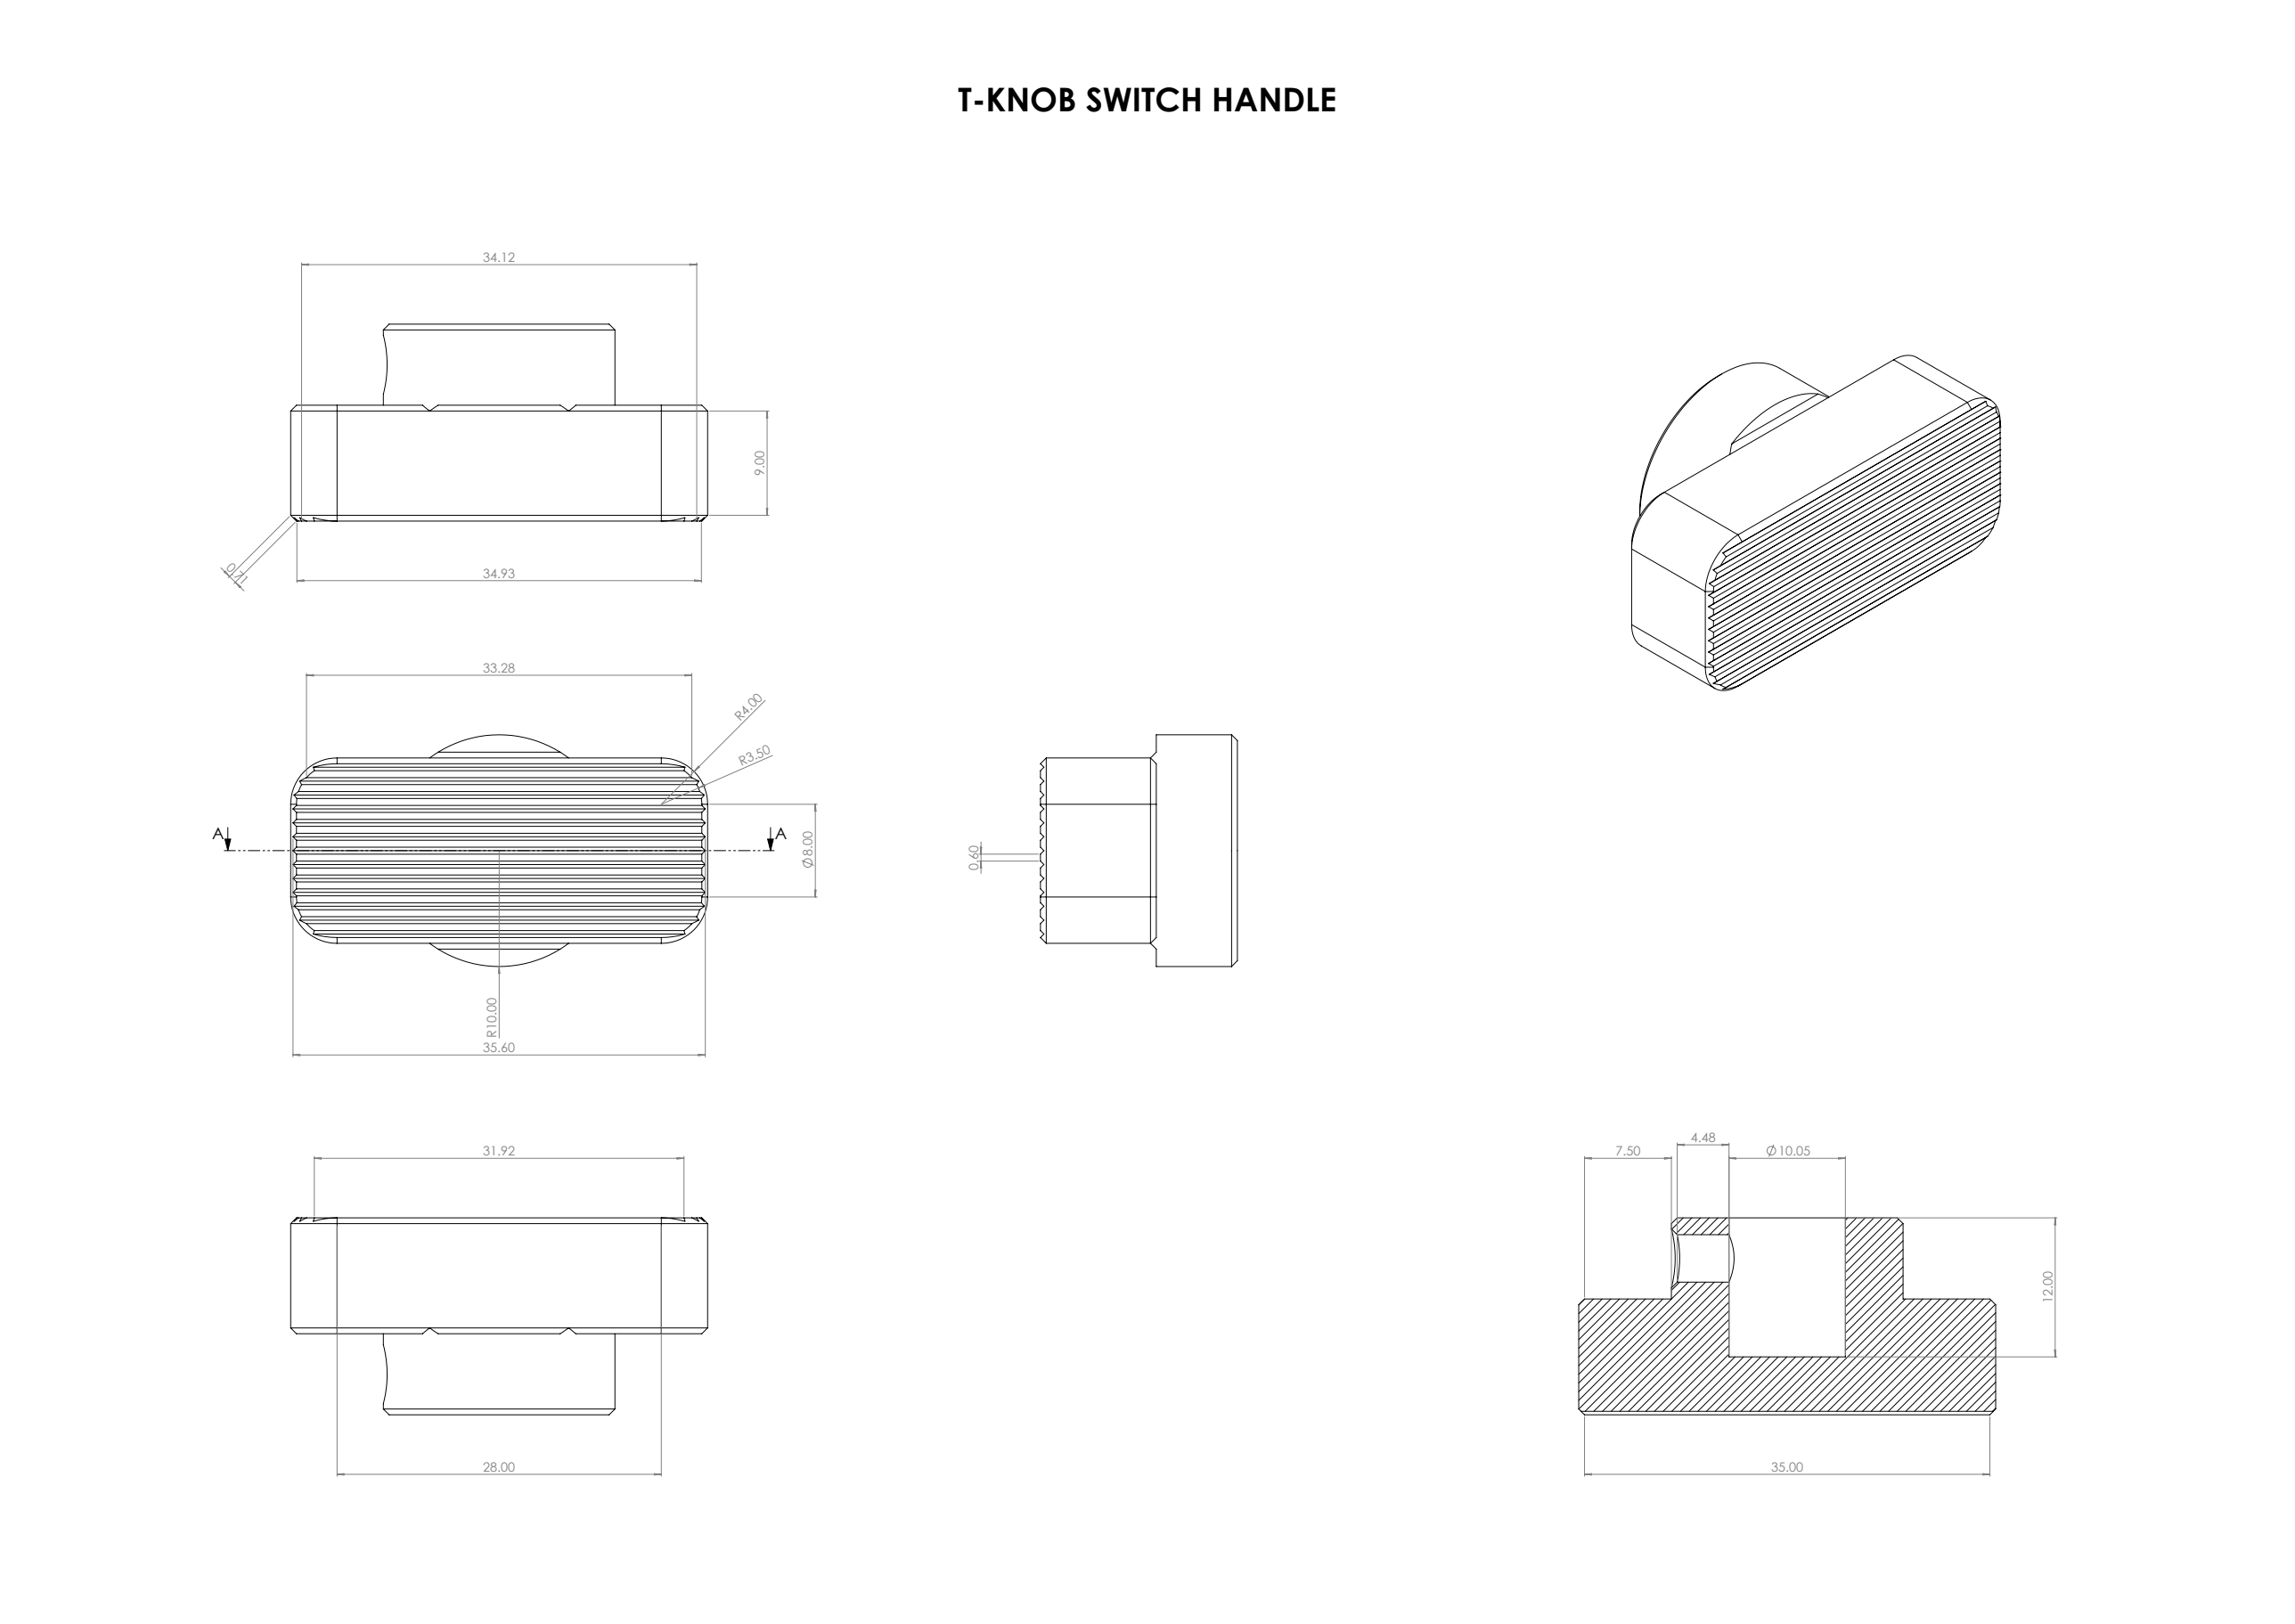
ISO-10303-21;
HEADER;
/* Generated by software containing ST-Developer
 * from STEP Tools, Inc. (www.steptools.com) 
 */

FILE_DESCRIPTION(
/* description */ (''),
/* implementation_level */ '2;1');

FILE_NAME(
/* name */ '09_T-Knob_Switch_Handle.step',
/* time_stamp */ '2026-10-21T01:59:45-07:00',
/* author */ (''),
/* organization */ (''),
/* preprocessor_version */ 'ST-DEVELOPER v20.2',
/* originating_system */ 'Autodesk Translation Framework v15.15.0.0',
/* authorisation */ '');

FILE_SCHEMA (('AUTOMOTIVE_DESIGN { 1 0 10303 214 3 1 1 }'));
ENDSEC;

DATA;
#10=MECHANICAL_DESIGN_GEOMETRIC_PRESENTATION_REPRESENTATION('',(#477),#18281);
#119=(
BOUNDED_CURVE()
B_SPLINE_CURVE(2,(#14814,#14815,#14816),.UNSPECIFIED.,.F.,.F.)
B_SPLINE_CURVE_WITH_KNOTS((3,3),(0.,0.0729284032695322),.UNSPECIFIED.)
CURVE()
GEOMETRIC_REPRESENTATION_ITEM()
RATIONAL_B_SPLINE_CURVE((1.,1.,1.))
REPRESENTATION_ITEM('')
);
#120=(
BOUNDED_CURVE()
B_SPLINE_CURVE(2,(#14820,#14821,#14822),.UNSPECIFIED.,.F.,.F.)
B_SPLINE_CURVE_WITH_KNOTS((3,3),(0.,0.072928403269532),.UNSPECIFIED.)
CURVE()
GEOMETRIC_REPRESENTATION_ITEM()
RATIONAL_B_SPLINE_CURVE((1.,1.,1.))
REPRESENTATION_ITEM('')
);
#121=(
BOUNDED_CURVE()
B_SPLINE_CURVE(2,(#14826,#14827,#14828),.UNSPECIFIED.,.F.,.F.)
B_SPLINE_CURVE_WITH_KNOTS((3,3),(0.,0.0457691166614135),.UNSPECIFIED.)
CURVE()
GEOMETRIC_REPRESENTATION_ITEM()
RATIONAL_B_SPLINE_CURVE((1.,1.,1.))
REPRESENTATION_ITEM('')
);
#122=(
BOUNDED_CURVE()
B_SPLINE_CURVE(2,(#14831,#14832,#14833),.UNSPECIFIED.,.F.,.F.)
B_SPLINE_CURVE_WITH_KNOTS((3,3),(0.,0.0457691166614134),.UNSPECIFIED.)
CURVE()
GEOMETRIC_REPRESENTATION_ITEM()
RATIONAL_B_SPLINE_CURVE((1.,1.,1.))
REPRESENTATION_ITEM('')
);
#123=(
BOUNDED_CURVE()
B_SPLINE_CURVE(2,(#14897,#14898,#14899),.UNSPECIFIED.,.F.,.F.)
B_SPLINE_CURVE_WITH_KNOTS((3,3),(0.,0.0577818255968905),.UNSPECIFIED.)
CURVE()
GEOMETRIC_REPRESENTATION_ITEM()
RATIONAL_B_SPLINE_CURVE((1.,1.,1.))
REPRESENTATION_ITEM('')
);
#124=(
BOUNDED_CURVE()
B_SPLINE_CURVE(2,(#14903,#14904,#14905),.UNSPECIFIED.,.F.,.F.)
B_SPLINE_CURVE_WITH_KNOTS((3,3),(0.,0.0577818255968905),.UNSPECIFIED.)
CURVE()
GEOMETRIC_REPRESENTATION_ITEM()
RATIONAL_B_SPLINE_CURVE((1.,1.,1.))
REPRESENTATION_ITEM('')
);
#125=(
BOUNDED_CURVE()
B_SPLINE_CURVE(2,(#14909,#14910,#14911),.UNSPECIFIED.,.F.,.F.)
B_SPLINE_CURVE_WITH_KNOTS((3,3),(0.,0.0492830096737056),.UNSPECIFIED.)
CURVE()
GEOMETRIC_REPRESENTATION_ITEM()
RATIONAL_B_SPLINE_CURVE((1.,1.,1.))
REPRESENTATION_ITEM('')
);
#126=(
BOUNDED_CURVE()
B_SPLINE_CURVE(2,(#14914,#14915,#14916),.UNSPECIFIED.,.F.,.F.)
B_SPLINE_CURVE_WITH_KNOTS((3,3),(0.,0.0492830096737056),.UNSPECIFIED.)
CURVE()
GEOMETRIC_REPRESENTATION_ITEM()
RATIONAL_B_SPLINE_CURVE((1.,1.,1.))
REPRESENTATION_ITEM('')
);
#127=(
BOUNDED_CURVE()
B_SPLINE_CURVE(2,(#14920,#14921,#14922),.UNSPECIFIED.,.F.,.F.)
B_SPLINE_CURVE_WITH_KNOTS((3,3),(0.,0.072928403269532),.UNSPECIFIED.)
CURVE()
GEOMETRIC_REPRESENTATION_ITEM()
RATIONAL_B_SPLINE_CURVE((1.,1.,1.))
REPRESENTATION_ITEM('')
);
#128=(
BOUNDED_CURVE()
B_SPLINE_CURVE(2,(#14926,#14927,#14928),.UNSPECIFIED.,.F.,.F.)
B_SPLINE_CURVE_WITH_KNOTS((3,3),(0.,0.0729284032695322),.UNSPECIFIED.)
CURVE()
GEOMETRIC_REPRESENTATION_ITEM()
RATIONAL_B_SPLINE_CURVE((1.,1.,1.))
REPRESENTATION_ITEM('')
);
#129=(
BOUNDED_CURVE()
B_SPLINE_CURVE(2,(#14932,#14933,#14934),.UNSPECIFIED.,.F.,.F.)
B_SPLINE_CURVE_WITH_KNOTS((3,3),(0.,0.0457691166614135),.UNSPECIFIED.)
CURVE()
GEOMETRIC_REPRESENTATION_ITEM()
RATIONAL_B_SPLINE_CURVE((1.,1.,1.))
REPRESENTATION_ITEM('')
);
#130=(
BOUNDED_CURVE()
B_SPLINE_CURVE(2,(#14937,#14938,#14939),.UNSPECIFIED.,.F.,.F.)
B_SPLINE_CURVE_WITH_KNOTS((3,3),(0.,0.0457691166614134),.UNSPECIFIED.)
CURVE()
GEOMETRIC_REPRESENTATION_ITEM()
RATIONAL_B_SPLINE_CURVE((1.,1.,1.))
REPRESENTATION_ITEM('')
);
#131=(
BOUNDED_CURVE()
B_SPLINE_CURVE(2,(#14973,#14974,#14975),.UNSPECIFIED.,.F.,.F.)
B_SPLINE_CURVE_WITH_KNOTS((3,3),(0.,0.210313307559557),.UNSPECIFIED.)
CURVE()
GEOMETRIC_REPRESENTATION_ITEM()
RATIONAL_B_SPLINE_CURVE((1.,1.,1.))
REPRESENTATION_ITEM('')
);
#132=(
BOUNDED_CURVE()
B_SPLINE_CURVE(2,(#14979,#14980,#14981),.UNSPECIFIED.,.F.,.F.)
B_SPLINE_CURVE_WITH_KNOTS((3,3),(0.210313307559557,0.420626615119114),
 .UNSPECIFIED.)
CURVE()
GEOMETRIC_REPRESENTATION_ITEM()
RATIONAL_B_SPLINE_CURVE((1.,1.,1.))
REPRESENTATION_ITEM('')
);
#133=(
BOUNDED_CURVE()
B_SPLINE_CURVE(2,(#14985,#14986,#14987),.UNSPECIFIED.,.F.,.F.)
B_SPLINE_CURVE_WITH_KNOTS((3,3),(0.,0.0433664286594662),.UNSPECIFIED.)
CURVE()
GEOMETRIC_REPRESENTATION_ITEM()
RATIONAL_B_SPLINE_CURVE((1.,1.,1.))
REPRESENTATION_ITEM('')
);
#134=(
BOUNDED_CURVE()
B_SPLINE_CURVE(2,(#14990,#14991,#14992),.UNSPECIFIED.,.F.,.F.)
B_SPLINE_CURVE_WITH_KNOTS((3,3),(0.,0.0433664286594663),.UNSPECIFIED.)
CURVE()
GEOMETRIC_REPRESENTATION_ITEM()
RATIONAL_B_SPLINE_CURVE((1.,1.,1.))
REPRESENTATION_ITEM('')
);
#135=(
BOUNDED_CURVE()
B_SPLINE_CURVE(2,(#15011,#15012,#15013),.UNSPECIFIED.,.F.,.F.)
B_SPLINE_CURVE_WITH_KNOTS((3,3),(0.,0.0577818255968905),.UNSPECIFIED.)
CURVE()
GEOMETRIC_REPRESENTATION_ITEM()
RATIONAL_B_SPLINE_CURVE((1.,1.,1.))
REPRESENTATION_ITEM('')
);
#136=(
BOUNDED_CURVE()
B_SPLINE_CURVE(2,(#15017,#15018,#15019),.UNSPECIFIED.,.F.,.F.)
B_SPLINE_CURVE_WITH_KNOTS((3,3),(0.,0.0577818255968905),.UNSPECIFIED.)
CURVE()
GEOMETRIC_REPRESENTATION_ITEM()
RATIONAL_B_SPLINE_CURVE((1.,1.,1.))
REPRESENTATION_ITEM('')
);
#137=(
BOUNDED_CURVE()
B_SPLINE_CURVE(2,(#15023,#15024,#15025),.UNSPECIFIED.,.F.,.F.)
B_SPLINE_CURVE_WITH_KNOTS((3,3),(0.,0.0492830096737056),.UNSPECIFIED.)
CURVE()
GEOMETRIC_REPRESENTATION_ITEM()
RATIONAL_B_SPLINE_CURVE((1.,1.,1.))
REPRESENTATION_ITEM('')
);
#138=(
BOUNDED_CURVE()
B_SPLINE_CURVE(2,(#15028,#15029,#15030),.UNSPECIFIED.,.F.,.F.)
B_SPLINE_CURVE_WITH_KNOTS((3,3),(0.,0.0492830096737056),.UNSPECIFIED.)
CURVE()
GEOMETRIC_REPRESENTATION_ITEM()
RATIONAL_B_SPLINE_CURVE((1.,1.,1.))
REPRESENTATION_ITEM('')
);
#139=(
BOUNDED_CURVE()
B_SPLINE_CURVE(2,(#15034,#15035,#15036),.UNSPECIFIED.,.F.,.F.)
B_SPLINE_CURVE_WITH_KNOTS((3,3),(0.,0.0433664286594662),.UNSPECIFIED.)
CURVE()
GEOMETRIC_REPRESENTATION_ITEM()
RATIONAL_B_SPLINE_CURVE((1.,1.,1.))
REPRESENTATION_ITEM('')
);
#140=(
BOUNDED_CURVE()
B_SPLINE_CURVE(2,(#15040,#15041,#15042),.UNSPECIFIED.,.F.,.F.)
B_SPLINE_CURVE_WITH_KNOTS((3,3),(0.,0.0433664286594662),.UNSPECIFIED.)
CURVE()
GEOMETRIC_REPRESENTATION_ITEM()
RATIONAL_B_SPLINE_CURVE((1.,1.,1.))
REPRESENTATION_ITEM('')
);
#141=(
BOUNDED_CURVE()
B_SPLINE_CURVE(2,(#15046,#15047,#15048),.UNSPECIFIED.,.F.,.F.)
B_SPLINE_CURVE_WITH_KNOTS((3,3),(0.210313307559558,0.420626615119116),
 .UNSPECIFIED.)
CURVE()
GEOMETRIC_REPRESENTATION_ITEM()
RATIONAL_B_SPLINE_CURVE((1.,1.,1.))
REPRESENTATION_ITEM('')
);
#142=(
BOUNDED_CURVE()
B_SPLINE_CURVE(2,(#15051,#15052,#15053),.UNSPECIFIED.,.F.,.F.)
B_SPLINE_CURVE_WITH_KNOTS((3,3),(0.,0.210313307559558),.UNSPECIFIED.)
CURVE()
GEOMETRIC_REPRESENTATION_ITEM()
RATIONAL_B_SPLINE_CURVE((1.,1.,1.))
REPRESENTATION_ITEM('')
);
#183=B_SPLINE_SURFACE_WITH_KNOTS('',3,3,((#14625,#14626,#14627,#14628,#14629,
#14630,#14631,#14632,#14633,#14634,#14635,#14636,#14637,#14638,#14639,#14640,
#14641,#14642,#14643,#14644),(#14645,#14646,#14647,#14648,#14649,#14650,
#14651,#14652,#14653,#14654,#14655,#14656,#14657,#14658,#14659,#14660,#14661,
#14662,#14663,#14664),(#14665,#14666,#14667,#14668,#14669,#14670,#14671,
#14672,#14673,#14674,#14675,#14676,#14677,#14678,#14679,#14680,#14681,#14682,
#14683,#14684),(#14685,#14686,#14687,#14688,#14689,#14690,#14691,#14692,
#14693,#14694,#14695,#14696,#14697,#14698,#14699,#14700,#14701,#14702,#14703,
#14704)),.UNSPECIFIED.,.F.,.T.,.F.,(4,4),(4,1,1,1,1,1,1,1,1,1,1,1,1,1,1,
1,1,4),(0.,1.),(0.929489890414013,1.01801273712011,1.06227416047316,1.10653558382621,
1.1950584305323,1.2835812772384,1.3721041239445,1.41636554729754,1.46062697065059,
1.54914981735669,1.63767266406279,1.68193408741583,1.72619551076888,1.81471835747498,
1.90324120418107,1.99176405088717,2.08028689759327,2.16880974429936),
 .UNSPECIFIED.);
#281=B_SPLINE_CURVE_WITH_KNOTS('',3,(#14708,#14709,#14710,#14711,#14712,
#14713,#14714,#14715,#14716,#14717,#14718,#14719,#14720,#14721,#14722,#14723,
#14724,#14725,#14726,#14727),.UNSPECIFIED.,.T.,.F.,(4,1,1,1,1,1,1,1,1,1,
1,1,1,1,1,1,1,4),(0.929489890414013,1.01801273712011,1.06227416047316,1.10653558382621,
1.1950584305323,1.2835812772384,1.3721041239445,1.41636554729754,1.46062697065059,
1.54914981735669,1.63767266406279,1.68193408741583,1.72619551076888,1.81471835747498,
1.90324120418107,1.99176405088717,2.08028689759327,2.16880974429936),
 .UNSPECIFIED.);
#282=B_SPLINE_CURVE_WITH_KNOTS('',3,(#14728,#14729,#14730,#14731,#14732,
#14733,#14734,#14735,#14736,#14737,#14738,#14739,#14740,#14741,#14742,#14743,
#14744,#14745,#14746,#14747),.UNSPECIFIED.,.T.,.F.,(4,1,1,1,1,1,1,1,1,1,
1,1,1,1,1,1,1,4),(-2.16880974429936,-2.08028689759327,-1.99176405088717,
-1.90324120418107,-1.81471835747498,-1.72619551076888,-1.68193408741583,
-1.63767266406279,-1.54914981735669,-1.46062697065059,-1.41636554729754,
-1.3721041239445,-1.2835812772384,-1.1950584305323,-1.10653558382621,-1.06227416047316,
-1.01801273712011,-0.929489890414013),.UNSPECIFIED.);
#283=B_SPLINE_CURVE_WITH_KNOTS('',3,(#14752,#14753,#14754,#14755,#14756,
#14757,#14758,#14759,#14760,#14761),.UNSPECIFIED.,.F.,.F.,(4,2,2,2,4),(0.,
0.0782650235733475,0.156530047146695,0.234708817404274,0.312887587661852),
 .UNSPECIFIED.);
#284=B_SPLINE_CURVE_WITH_KNOTS('',3,(#14762,#14763,#14764,#14765,#14766,
#14767,#14768,#14769,#14770,#14771,#14772,#14773,#14774,#14775,#14776,#14777,
#14778,#14779,#14780,#14781,#14782,#14783,#14784,#14785,#14786,#14787),
 .UNSPECIFIED.,.F.,.F.,(4,2,2,2,2,2,2,2,2,2,2,2,4),(0.312887587661852,0.391066357919431,
0.469245128177009,0.547510151750357,0.625775175323705,0.704040198897052,
0.782305222470399,0.860483992727978,0.938662762985557,1.01684153324314,
1.09502030350071,1.17328532707406,1.25155035064741),.UNSPECIFIED.);
#421=CONICAL_SURFACE('',#9730,3.75,0.785398163397447);
#422=CONICAL_SURFACE('',#9738,3.75,0.785398163397447);
#423=CONICAL_SURFACE('',#9741,3.75,0.785398163397447);
#424=CONICAL_SURFACE('',#9748,3.75,0.785398163397447);
#425=CONICAL_SURFACE('',#9792,3.75,0.785398163397448);
#426=CONICAL_SURFACE('',#9816,3.75,0.785398163397447);
#427=CONICAL_SURFACE('',#9831,3.75,0.785398163397447);
#428=CONICAL_SURFACE('',#9834,3.75,0.785398163397448);
#429=CONICAL_SURFACE('',#9846,9.75,0.785398163397449);
#446=SHAPE_REPRESENTATION_RELATIONSHIP('SRR','None',#18348,#459);
#459=ADVANCED_BREP_SHAPE_REPRESENTATION('',(#490),#18277);
#477=STYLED_ITEM('',(#18488),#490);
#490=MANIFOLD_SOLID_BREP('Body1',#9094);
#533=CYLINDRICAL_SURFACE('',#9752,2.05);
#534=CYLINDRICAL_SURFACE('',#9753,10.);
#535=CYLINDRICAL_SURFACE('',#9823,4.);
#536=CYLINDRICAL_SURFACE('',#9825,4.);
#537=CYLINDRICAL_SURFACE('',#9828,4.);
#538=CYLINDRICAL_SURFACE('',#9838,4.);
#539=CYLINDRICAL_SURFACE('',#9842,5.025);
#623=FACE_BOUND('',#1792,.T.);
#624=FACE_BOUND('',#1855,.T.);
#625=FACE_BOUND('',#1857,.T.);
#763=CIRCLE('',#9731,4.);
#764=CIRCLE('',#9732,3.5);
#765=CIRCLE('',#9736,3.5);
#766=CIRCLE('',#9737,10.);
#767=CIRCLE('',#9739,4.);
#768=CIRCLE('',#9742,4.);
#769=CIRCLE('',#9743,3.5);
#770=CIRCLE('',#9746,10.);
#771=CIRCLE('',#9747,3.5);
#772=CIRCLE('',#9749,4.);
#773=CIRCLE('',#9757,10.);
#774=CIRCLE('',#9758,10.);
#775=CIRCLE('',#9759,10.);
#776=CIRCLE('',#9763,10.);
#777=CIRCLE('',#9765,5.025);
#778=CIRCLE('',#9793,3.5);
#779=CIRCLE('',#9794,4.);
#780=CIRCLE('',#9795,3.5);
#781=CIRCLE('',#9796,3.5);
#782=CIRCLE('',#9799,3.5);
#783=CIRCLE('',#9800,3.5);
#784=CIRCLE('',#9802,3.5);
#785=CIRCLE('',#9803,3.5);
#786=CIRCLE('',#9807,3.5);
#787=CIRCLE('',#9809,3.5);
#788=CIRCLE('',#9811,3.5);
#789=CIRCLE('',#9817,4.);
#790=CIRCLE('',#9818,3.5);
#791=CIRCLE('',#9826,4.);
#792=CIRCLE('',#9829,4.);
#793=CIRCLE('',#9835,3.5);
#794=CIRCLE('',#9843,5.025);
#795=CIRCLE('',#9845,9.5);
#834=ELLIPSE('',#9734,14.142135623731,10.);
#835=ELLIPSE('',#9751,14.142135623731,10.);
#836=ELLIPSE('',#9754,14.142135623731,10.);
#837=ELLIPSE('',#9755,14.142135623731,10.);
#838=ELLIPSE('',#9756,14.142135623731,10.);
#839=ELLIPSE('',#9760,14.142135623731,10.);
#840=ELLIPSE('',#9761,14.142135623731,10.);
#841=ELLIPSE('',#9762,14.142135623731,10.);
#1213=FACE_OUTER_BOUND('',#1779,.T.);
#1214=FACE_OUTER_BOUND('',#1780,.T.);
#1215=FACE_OUTER_BOUND('',#1781,.T.);
#1216=FACE_OUTER_BOUND('',#1782,.T.);
#1217=FACE_OUTER_BOUND('',#1783,.T.);
#1218=FACE_OUTER_BOUND('',#1784,.T.);
#1219=FACE_OUTER_BOUND('',#1785,.T.);
#1220=FACE_OUTER_BOUND('',#1786,.T.);
#1221=FACE_OUTER_BOUND('',#1787,.T.);
#1222=FACE_OUTER_BOUND('',#1788,.T.);
#1223=FACE_OUTER_BOUND('',#1789,.T.);
#1224=FACE_OUTER_BOUND('',#1790,.T.);
#1225=FACE_OUTER_BOUND('',#1791,.T.);
#1226=FACE_OUTER_BOUND('',#1793,.T.);
#1227=FACE_OUTER_BOUND('',#1794,.T.);
#1228=FACE_OUTER_BOUND('',#1795,.T.);
#1229=FACE_OUTER_BOUND('',#1796,.T.);
#1230=FACE_OUTER_BOUND('',#1797,.T.);
#1231=FACE_OUTER_BOUND('',#1798,.T.);
#1232=FACE_OUTER_BOUND('',#1799,.T.);
#1233=FACE_OUTER_BOUND('',#1800,.T.);
#1234=FACE_OUTER_BOUND('',#1801,.T.);
#1235=FACE_OUTER_BOUND('',#1802,.T.);
#1236=FACE_OUTER_BOUND('',#1803,.T.);
#1237=FACE_OUTER_BOUND('',#1804,.T.);
#1238=FACE_OUTER_BOUND('',#1805,.T.);
#1239=FACE_OUTER_BOUND('',#1806,.T.);
#1240=FACE_OUTER_BOUND('',#1807,.T.);
#1241=FACE_OUTER_BOUND('',#1808,.T.);
#1242=FACE_OUTER_BOUND('',#1809,.T.);
#1243=FACE_OUTER_BOUND('',#1810,.T.);
#1244=FACE_OUTER_BOUND('',#1811,.T.);
#1245=FACE_OUTER_BOUND('',#1812,.T.);
#1246=FACE_OUTER_BOUND('',#1813,.T.);
#1247=FACE_OUTER_BOUND('',#1814,.T.);
#1248=FACE_OUTER_BOUND('',#1815,.T.);
#1249=FACE_OUTER_BOUND('',#1816,.T.);
#1250=FACE_OUTER_BOUND('',#1817,.T.);
#1251=FACE_OUTER_BOUND('',#1818,.T.);
#1252=FACE_OUTER_BOUND('',#1819,.T.);
#1253=FACE_OUTER_BOUND('',#1820,.T.);
#1254=FACE_OUTER_BOUND('',#1821,.T.);
#1255=FACE_OUTER_BOUND('',#1822,.T.);
#1256=FACE_OUTER_BOUND('',#1823,.T.);
#1257=FACE_OUTER_BOUND('',#1824,.T.);
#1258=FACE_OUTER_BOUND('',#1825,.T.);
#1259=FACE_OUTER_BOUND('',#1826,.T.);
#1260=FACE_OUTER_BOUND('',#1827,.T.);
#1261=FACE_OUTER_BOUND('',#1828,.T.);
#1262=FACE_OUTER_BOUND('',#1829,.T.);
#1263=FACE_OUTER_BOUND('',#1830,.T.);
#1264=FACE_OUTER_BOUND('',#1831,.T.);
#1265=FACE_OUTER_BOUND('',#1832,.T.);
#1266=FACE_OUTER_BOUND('',#1833,.T.);
#1267=FACE_OUTER_BOUND('',#1834,.T.);
#1268=FACE_OUTER_BOUND('',#1835,.T.);
#1269=FACE_OUTER_BOUND('',#1836,.T.);
#1270=FACE_OUTER_BOUND('',#1837,.T.);
#1271=FACE_OUTER_BOUND('',#1838,.T.);
#1272=FACE_OUTER_BOUND('',#1839,.T.);
#1273=FACE_OUTER_BOUND('',#1840,.T.);
#1274=FACE_OUTER_BOUND('',#1841,.T.);
#1275=FACE_OUTER_BOUND('',#1842,.T.);
#1276=FACE_OUTER_BOUND('',#1843,.T.);
#1277=FACE_OUTER_BOUND('',#1844,.T.);
#1278=FACE_OUTER_BOUND('',#1845,.T.);
#1279=FACE_OUTER_BOUND('',#1846,.T.);
#1280=FACE_OUTER_BOUND('',#1847,.T.);
#1281=FACE_OUTER_BOUND('',#1848,.T.);
#1282=FACE_OUTER_BOUND('',#1849,.T.);
#1283=FACE_OUTER_BOUND('',#1850,.T.);
#1284=FACE_OUTER_BOUND('',#1851,.T.);
#1285=FACE_OUTER_BOUND('',#1852,.T.);
#1286=FACE_OUTER_BOUND('',#1853,.T.);
#1287=FACE_OUTER_BOUND('',#1854,.T.);
#1288=FACE_OUTER_BOUND('',#1856,.T.);
#1289=FACE_OUTER_BOUND('',#1858,.T.);
#1779=EDGE_LOOP('',(#7464,#7465,#7466,#7467));
#1780=EDGE_LOOP('',(#7468,#7469,#7470,#7471));
#1781=EDGE_LOOP('',(#7472,#7473,#7474,#7475,#7476,#7477));
#1782=EDGE_LOOP('',(#7478,#7479,#7480,#7481));
#1783=EDGE_LOOP('',(#7482,#7483,#7484,#7485));
#1784=EDGE_LOOP('',(#7486,#7487,#7488,#7489));
#1785=EDGE_LOOP('',(#7490,#7491,#7492,#7493));
#1786=EDGE_LOOP('',(#7494,#7495,#7496,#7497,#7498,#7499));
#1787=EDGE_LOOP('',(#7500,#7501,#7502,#7503));
#1788=EDGE_LOOP('',(#7504,#7505,#7506,#7507));
#1789=EDGE_LOOP('',(#7508,#7509,#7510,#7511));
#1790=EDGE_LOOP('',(#7512,#7513,#7514,#7515,#7516));
#1791=EDGE_LOOP('',(#7517,#7518,#7519,#7520,#7521,#7522,#7523,#7524,#7525,
#7526,#7527,#7528,#7529,#7530,#7531,#7532));
#1792=EDGE_LOOP('',(#7533));
#1793=EDGE_LOOP('',(#7534));
#1794=EDGE_LOOP('',(#7535,#7536,#7537,#7538));
#1795=EDGE_LOOP('',(#7539,#7540,#7541,#7542));
#1796=EDGE_LOOP('',(#7543,#7544,#7545,#7546));
#1797=EDGE_LOOP('',(#7547,#7548,#7549,#7550));
#1798=EDGE_LOOP('',(#7551,#7552,#7553,#7554));
#1799=EDGE_LOOP('',(#7555,#7556,#7557,#7558));
#1800=EDGE_LOOP('',(#7559,#7560,#7561,#7562));
#1801=EDGE_LOOP('',(#7563,#7564,#7565,#7566));
#1802=EDGE_LOOP('',(#7567,#7568,#7569,#7570));
#1803=EDGE_LOOP('',(#7571,#7572,#7573,#7574));
#1804=EDGE_LOOP('',(#7575,#7576,#7577,#7578));
#1805=EDGE_LOOP('',(#7579,#7580,#7581,#7582));
#1806=EDGE_LOOP('',(#7583,#7584,#7585,#7586));
#1807=EDGE_LOOP('',(#7587,#7588,#7589,#7590));
#1808=EDGE_LOOP('',(#7591,#7592,#7593,#7594));
#1809=EDGE_LOOP('',(#7595,#7596,#7597,#7598));
#1810=EDGE_LOOP('',(#7599,#7600,#7601,#7602));
#1811=EDGE_LOOP('',(#7603,#7604,#7605,#7606));
#1812=EDGE_LOOP('',(#7607,#7608,#7609,#7610));
#1813=EDGE_LOOP('',(#7611,#7612,#7613,#7614));
#1814=EDGE_LOOP('',(#7615,#7616,#7617,#7618));
#1815=EDGE_LOOP('',(#7619,#7620,#7621,#7622));
#1816=EDGE_LOOP('',(#7623,#7624,#7625,#7626));
#1817=EDGE_LOOP('',(#7627,#7628,#7629,#7630));
#1818=EDGE_LOOP('',(#7631,#7632,#7633,#7634));
#1819=EDGE_LOOP('',(#7635,#7636,#7637,#7638));
#1820=EDGE_LOOP('',(#7639,#7640,#7641,#7642,#7643,#7644,#7645,#7646,#7647,
#7648,#7649,#7650));
#1821=EDGE_LOOP('',(#7651,#7652,#7653,#7654,#7655,#7656,#7657,#7658,#7659,
#7660,#7661,#7662,#7663,#7664,#7665,#7666,#7667,#7668,#7669,#7670,#7671,
#7672,#7673,#7674,#7675));
#1822=EDGE_LOOP('',(#7676,#7677,#7678,#7679));
#1823=EDGE_LOOP('',(#7680,#7681,#7682,#7683,#7684,#7685));
#1824=EDGE_LOOP('',(#7686,#7687,#7688,#7689));
#1825=EDGE_LOOP('',(#7690,#7691,#7692,#7693));
#1826=EDGE_LOOP('',(#7694,#7695,#7696,#7697));
#1827=EDGE_LOOP('',(#7698,#7699,#7700,#7701));
#1828=EDGE_LOOP('',(#7702,#7703,#7704,#7705,#7706,#7707));
#1829=EDGE_LOOP('',(#7708,#7709,#7710,#7711));
#1830=EDGE_LOOP('',(#7712,#7713,#7714,#7715));
#1831=EDGE_LOOP('',(#7716,#7717,#7718,#7719));
#1832=EDGE_LOOP('',(#7720,#7721,#7722,#7723));
#1833=EDGE_LOOP('',(#7724,#7725,#7726,#7727,#7728,#7729,#7730,#7731,#7732,
#7733,#7734,#7735));
#1834=EDGE_LOOP('',(#7736,#7737,#7738,#7739));
#1835=EDGE_LOOP('',(#7740,#7741,#7742,#7743,#7744,#7745));
#1836=EDGE_LOOP('',(#7746,#7747,#7748,#7749));
#1837=EDGE_LOOP('',(#7750,#7751,#7752,#7753,#7754,#7755));
#1838=EDGE_LOOP('',(#7756,#7757,#7758,#7759));
#1839=EDGE_LOOP('',(#7760,#7761,#7762,#7763));
#1840=EDGE_LOOP('',(#7764,#7765,#7766,#7767));
#1841=EDGE_LOOP('',(#7768,#7769,#7770,#7771));
#1842=EDGE_LOOP('',(#7772,#7773,#7774,#7775));
#1843=EDGE_LOOP('',(#7776,#7777,#7778,#7779));
#1844=EDGE_LOOP('',(#7780,#7781,#7782,#7783,#7784,#7785,#7786,#7787,#7788,
#7789,#7790,#7791));
#1845=EDGE_LOOP('',(#7792,#7793,#7794,#7795));
#1846=EDGE_LOOP('',(#7796,#7797,#7798,#7799));
#1847=EDGE_LOOP('',(#7800,#7801,#7802,#7803,#7804,#7805,#7806,#7807,#7808,
#7809,#7810,#7811));
#1848=EDGE_LOOP('',(#7812,#7813,#7814,#7815,#7816,#7817,#7818,#7819,#7820,
#7821,#7822,#7823,#7824,#7825,#7826,#7827,#7828,#7829,#7830,#7831,#7832,
#7833,#7834,#7835,#7836));
#1849=EDGE_LOOP('',(#7837,#7838,#7839,#7840));
#1850=EDGE_LOOP('',(#7841,#7842,#7843,#7844));
#1851=EDGE_LOOP('',(#7845,#7846,#7847,#7848));
#1852=EDGE_LOOP('',(#7849,#7850,#7851));
#1853=EDGE_LOOP('',(#7852,#7853));
#1854=EDGE_LOOP('',(#7854,#7855,#7856,#7857));
#1855=EDGE_LOOP('',(#7858,#7859));
#1856=EDGE_LOOP('',(#7860));
#1857=EDGE_LOOP('',(#7861));
#1858=EDGE_LOOP('',(#7862,#7863,#7864,#7865));
#2571=LINE('',#14566,#3416);
#2572=LINE('',#14570,#3417);
#2573=LINE('',#14574,#3418);
#2574=LINE('',#14577,#3419);
#2575=LINE('',#14580,#3420);
#2576=LINE('',#14584,#3421);
#2577=LINE('',#14588,#3422);
#2578=LINE('',#14591,#3423);
#2579=LINE('',#14593,#3424);
#2580=LINE('',#14597,#3425);
#2581=LINE('',#14601,#3426);
#2582=LINE('',#14605,#3427);
#2583=LINE('',#14607,#3428);
#2584=LINE('',#14608,#3429);
#2585=LINE('',#14611,#3430);
#2586=LINE('',#14615,#3431);
#2587=LINE('',#14619,#3432);
#2588=LINE('',#14624,#3433);
#2589=LINE('',#14707,#3434);
#2590=LINE('',#14750,#3435);
#2591=LINE('',#14798,#3436);
#2592=LINE('',#14818,#3437);
#2593=LINE('',#14823,#3438);
#2594=LINE('',#14830,#3439);
#2595=LINE('',#14837,#3440);
#2596=LINE('',#14839,#3441);
#2597=LINE('',#14841,#3442);
#2598=LINE('',#14842,#3443);
#2599=LINE('',#14845,#3444);
#2600=LINE('',#14847,#3445);
#2601=LINE('',#14848,#3446);
#2602=LINE('',#14852,#3447);
#2603=LINE('',#14854,#3448);
#2604=LINE('',#14856,#3449);
#2605=LINE('',#14857,#3450);
#2606=LINE('',#14860,#3451);
#2607=LINE('',#14862,#3452);
#2608=LINE('',#14863,#3453);
#2609=LINE('',#14867,#3454);
#2610=LINE('',#14869,#3455);
#2611=LINE('',#14871,#3456);
#2612=LINE('',#14872,#3457);
#2613=LINE('',#14875,#3458);
#2614=LINE('',#14877,#3459);
#2615=LINE('',#14878,#3460);
#2616=LINE('',#14882,#3461);
#2617=LINE('',#14884,#3462);
#2618=LINE('',#14886,#3463);
#2619=LINE('',#14887,#3464);
#2620=LINE('',#14890,#3465);
#2621=LINE('',#14892,#3466);
#2622=LINE('',#14893,#3467);
#2623=LINE('',#14901,#3468);
#2624=LINE('',#14906,#3469);
#2625=LINE('',#14913,#3470);
#2626=LINE('',#14924,#3471);
#2627=LINE('',#14929,#3472);
#2628=LINE('',#14936,#3473);
#2629=LINE('',#14943,#3474);
#2630=LINE('',#14945,#3475);
#2631=LINE('',#14947,#3476);
#2632=LINE('',#14948,#3477);
#2633=LINE('',#14951,#3478);
#2634=LINE('',#14953,#3479);
#2635=LINE('',#14954,#3480);
#2636=LINE('',#14958,#3481);
#2637=LINE('',#14960,#3482);
#2638=LINE('',#14962,#3483);
#2639=LINE('',#14963,#3484);
#2640=LINE('',#14966,#3485);
#2641=LINE('',#14968,#3486);
#2642=LINE('',#14969,#3487);
#2643=LINE('',#14977,#3488);
#2644=LINE('',#14982,#3489);
#2645=LINE('',#14989,#3490);
#2646=LINE('',#14996,#3491);
#2647=LINE('',#14998,#3492);
#2648=LINE('',#15000,#3493);
#2649=LINE('',#15001,#3494);
#2650=LINE('',#15004,#3495);
#2651=LINE('',#15006,#3496);
#2652=LINE('',#15007,#3497);
#2653=LINE('',#15015,#3498);
#2654=LINE('',#15020,#3499);
#2655=LINE('',#15027,#3500);
#2656=LINE('',#15038,#3501);
#2657=LINE('',#15043,#3502);
#2658=LINE('',#15050,#3503);
#2659=LINE('',#15058,#3504);
#2660=LINE('',#15061,#3505);
#2661=LINE('',#15066,#3506);
#2662=LINE('',#15068,#3507);
#2663=LINE('',#15069,#3508);
#2664=LINE('',#15070,#3509);
#2665=LINE('',#15071,#3510);
#2666=LINE('',#15072,#3511);
#2667=LINE('',#15073,#3512);
#2668=LINE('',#15074,#3513);
#2669=LINE('',#15075,#3514);
#2670=LINE('',#15076,#3515);
#2671=LINE('',#15082,#3516);
#2672=LINE('',#15086,#3517);
#2673=LINE('',#15088,#3518);
#2674=LINE('',#15096,#3519);
#2675=LINE('',#15098,#3520);
#2676=LINE('',#15100,#3521);
#2677=LINE('',#15102,#3522);
#2678=LINE('',#15104,#3523);
#2679=LINE('',#15107,#3524);
#2680=LINE('',#15111,#3525);
#2681=LINE('',#15112,#3526);
#2682=LINE('',#15114,#3527);
#2683=LINE('',#15116,#3528);
#2684=LINE('',#15117,#3529);
#2685=LINE('',#15118,#3530);
#2686=LINE('',#15120,#3531);
#2687=LINE('',#15121,#3532);
#2688=LINE('',#15123,#3533);
#2689=LINE('',#15124,#3534);
#2690=LINE('',#15126,#3535);
#2691=LINE('',#15127,#3536);
#2692=LINE('',#15129,#3537);
#2693=LINE('',#15133,#3538);
#2694=LINE('',#15139,#3539);
#2695=LINE('',#15141,#3540);
#2696=LINE('',#15143,#3541);
#2697=LINE('',#15144,#3542);
#2698=LINE('',#15147,#3543);
#2699=LINE('',#15150,#3544);
#2700=LINE('',#15154,#3545);
#2701=LINE('',#15160,#3546);
#2702=LINE('',#15166,#3547);
#3416=VECTOR('',#11583,10.);
#3417=VECTOR('',#11586,10.);
#3418=VECTOR('',#11591,10.);
#3419=VECTOR('',#11594,10.);
#3420=VECTOR('',#11597,10.);
#3421=VECTOR('',#11600,10.);
#3422=VECTOR('',#11605,10.);
#3423=VECTOR('',#11608,10.);
#3424=VECTOR('',#11611,10.);
#3425=VECTOR('',#11614,10.);
#3426=VECTOR('',#11617,10.);
#3427=VECTOR('',#11622,10.);
#3428=VECTOR('',#11623,10.);
#3429=VECTOR('',#11624,10.);
#3430=VECTOR('',#11627,10.);
#3431=VECTOR('',#11630,10.);
#3432=VECTOR('',#11635,10.);
#3433=VECTOR('',#11642,10.);
#3434=VECTOR('',#11643,10.);
#3435=VECTOR('',#11646,2.05);
#3436=VECTOR('',#11657,10.);
#3437=VECTOR('',#11676,10.);
#3438=VECTOR('',#11677,10.);
#3439=VECTOR('',#11680,10.);
#3440=VECTOR('',#11683,10.);
#3441=VECTOR('',#11684,10.);
#3442=VECTOR('',#11685,10.);
#3443=VECTOR('',#11686,10.);
#3444=VECTOR('',#11689,10.);
#3445=VECTOR('',#11690,10.);
#3446=VECTOR('',#11691,10.);
#3447=VECTOR('',#11694,10.);
#3448=VECTOR('',#11695,10.);
#3449=VECTOR('',#11696,10.);
#3450=VECTOR('',#11697,10.);
#3451=VECTOR('',#11700,10.);
#3452=VECTOR('',#11701,10.);
#3453=VECTOR('',#11702,10.);
#3454=VECTOR('',#11705,10.);
#3455=VECTOR('',#11706,10.);
#3456=VECTOR('',#11707,10.);
#3457=VECTOR('',#11708,10.);
#3458=VECTOR('',#11711,10.);
#3459=VECTOR('',#11712,10.);
#3460=VECTOR('',#11713,10.);
#3461=VECTOR('',#11716,10.);
#3462=VECTOR('',#11717,10.);
#3463=VECTOR('',#11718,10.);
#3464=VECTOR('',#11719,10.);
#3465=VECTOR('',#11722,10.);
#3466=VECTOR('',#11723,10.);
#3467=VECTOR('',#11724,10.);
#3468=VECTOR('',#11727,10.);
#3469=VECTOR('',#11728,10.);
#3470=VECTOR('',#11731,10.);
#3471=VECTOR('',#11734,10.);
#3472=VECTOR('',#11735,10.);
#3473=VECTOR('',#11738,10.);
#3474=VECTOR('',#11741,10.);
#3475=VECTOR('',#11742,10.);
#3476=VECTOR('',#11743,10.);
#3477=VECTOR('',#11744,10.);
#3478=VECTOR('',#11747,10.);
#3479=VECTOR('',#11748,10.);
#3480=VECTOR('',#11749,10.);
#3481=VECTOR('',#11752,10.);
#3482=VECTOR('',#11753,10.);
#3483=VECTOR('',#11754,10.);
#3484=VECTOR('',#11755,10.);
#3485=VECTOR('',#11758,10.);
#3486=VECTOR('',#11759,10.);
#3487=VECTOR('',#11760,10.);
#3488=VECTOR('',#11763,10.);
#3489=VECTOR('',#11764,10.);
#3490=VECTOR('',#11767,10.);
#3491=VECTOR('',#11770,10.);
#3492=VECTOR('',#11771,10.);
#3493=VECTOR('',#11772,10.);
#3494=VECTOR('',#11773,10.);
#3495=VECTOR('',#11776,10.);
#3496=VECTOR('',#11777,10.);
#3497=VECTOR('',#11778,10.);
#3498=VECTOR('',#11781,10.);
#3499=VECTOR('',#11782,10.);
#3500=VECTOR('',#11785,10.);
#3501=VECTOR('',#11788,10.);
#3502=VECTOR('',#11789,10.);
#3503=VECTOR('',#11792,10.);
#3504=VECTOR('',#11797,10.);
#3505=VECTOR('',#11800,10.);
#3506=VECTOR('',#11807,10.);
#3507=VECTOR('',#11808,10.);
#3508=VECTOR('',#11809,10.);
#3509=VECTOR('',#11810,10.);
#3510=VECTOR('',#11811,10.);
#3511=VECTOR('',#11812,10.);
#3512=VECTOR('',#11813,10.);
#3513=VECTOR('',#11814,10.);
#3514=VECTOR('',#11815,10.);
#3515=VECTOR('',#11816,10.);
#3516=VECTOR('',#11825,10.);
#3517=VECTOR('',#11832,10.);
#3518=VECTOR('',#11835,10.);
#3519=VECTOR('',#11848,10.);
#3520=VECTOR('',#11851,10.);
#3521=VECTOR('',#11854,10.);
#3522=VECTOR('',#11857,10.);
#3523=VECTOR('',#11860,10.);
#3524=VECTOR('',#11863,10.);
#3525=VECTOR('',#11870,10.);
#3526=VECTOR('',#11871,10.);
#3527=VECTOR('',#11874,10.);
#3528=VECTOR('',#11875,10.);
#3529=VECTOR('',#11876,10.);
#3530=VECTOR('',#11877,10.);
#3531=VECTOR('',#11880,10.);
#3532=VECTOR('',#11881,10.);
#3533=VECTOR('',#11884,10.);
#3534=VECTOR('',#11885,10.);
#3535=VECTOR('',#11886,10.);
#3536=VECTOR('',#11887,10.);
#3537=VECTOR('',#11890,10.);
#3538=VECTOR('',#11895,10.);
#3539=VECTOR('',#11904,10.);
#3540=VECTOR('',#11907,10.);
#3541=VECTOR('',#11910,10.);
#3542=VECTOR('',#11911,10.);
#3543=VECTOR('',#11916,10.);
#3544=VECTOR('',#11921,10.);
#3545=VECTOR('',#11928,10.);
#3546=VECTOR('',#11937,5.025);
#3547=VECTOR('',#11946,9.75);
#4169=VERTEX_POINT('',#14564);
#4170=VERTEX_POINT('',#14565);
#4171=VERTEX_POINT('',#14567);
#4172=VERTEX_POINT('',#14569);
#4173=VERTEX_POINT('',#14573);
#4174=VERTEX_POINT('',#14575);
#4175=VERTEX_POINT('',#14579);
#4176=VERTEX_POINT('',#14581);
#4177=VERTEX_POINT('',#14583);
#4178=VERTEX_POINT('',#14587);
#4179=VERTEX_POINT('',#14589);
#4180=VERTEX_POINT('',#14595);
#4181=VERTEX_POINT('',#14596);
#4182=VERTEX_POINT('',#14598);
#4183=VERTEX_POINT('',#14600);
#4184=VERTEX_POINT('',#14604);
#4185=VERTEX_POINT('',#14606);
#4186=VERTEX_POINT('',#14610);
#4187=VERTEX_POINT('',#14612);
#4188=VERTEX_POINT('',#14614);
#4189=VERTEX_POINT('',#14618);
#4190=VERTEX_POINT('',#14622);
#4191=VERTEX_POINT('',#14705);
#4192=VERTEX_POINT('',#14706);
#4193=VERTEX_POINT('',#14749);
#4194=VERTEX_POINT('',#14751);
#4195=VERTEX_POINT('',#14789);
#4196=VERTEX_POINT('',#14791);
#4197=VERTEX_POINT('',#14793);
#4198=VERTEX_POINT('',#14795);
#4199=VERTEX_POINT('',#14797);
#4200=VERTEX_POINT('',#14800);
#4201=VERTEX_POINT('',#14803);
#4202=VERTEX_POINT('',#14805);
#4203=VERTEX_POINT('',#14809);
#4204=VERTEX_POINT('',#14812);
#4205=VERTEX_POINT('',#14813);
#4206=VERTEX_POINT('',#14817);
#4207=VERTEX_POINT('',#14819);
#4208=VERTEX_POINT('',#14825);
#4209=VERTEX_POINT('',#14829);
#4210=VERTEX_POINT('',#14835);
#4211=VERTEX_POINT('',#14836);
#4212=VERTEX_POINT('',#14838);
#4213=VERTEX_POINT('',#14840);
#4214=VERTEX_POINT('',#14844);
#4215=VERTEX_POINT('',#14846);
#4216=VERTEX_POINT('',#14850);
#4217=VERTEX_POINT('',#14851);
#4218=VERTEX_POINT('',#14853);
#4219=VERTEX_POINT('',#14855);
#4220=VERTEX_POINT('',#14859);
#4221=VERTEX_POINT('',#14861);
#4222=VERTEX_POINT('',#14865);
#4223=VERTEX_POINT('',#14866);
#4224=VERTEX_POINT('',#14868);
#4225=VERTEX_POINT('',#14870);
#4226=VERTEX_POINT('',#14874);
#4227=VERTEX_POINT('',#14876);
#4228=VERTEX_POINT('',#14880);
#4229=VERTEX_POINT('',#14881);
#4230=VERTEX_POINT('',#14883);
#4231=VERTEX_POINT('',#14885);
#4232=VERTEX_POINT('',#14889);
#4233=VERTEX_POINT('',#14891);
#4234=VERTEX_POINT('',#14895);
#4235=VERTEX_POINT('',#14896);
#4236=VERTEX_POINT('',#14900);
#4237=VERTEX_POINT('',#14902);
#4238=VERTEX_POINT('',#14908);
#4239=VERTEX_POINT('',#14912);
#4240=VERTEX_POINT('',#14918);
#4241=VERTEX_POINT('',#14919);
#4242=VERTEX_POINT('',#14923);
#4243=VERTEX_POINT('',#14925);
#4244=VERTEX_POINT('',#14931);
#4245=VERTEX_POINT('',#14935);
#4246=VERTEX_POINT('',#14941);
#4247=VERTEX_POINT('',#14942);
#4248=VERTEX_POINT('',#14944);
#4249=VERTEX_POINT('',#14946);
#4250=VERTEX_POINT('',#14950);
#4251=VERTEX_POINT('',#14952);
#4252=VERTEX_POINT('',#14956);
#4253=VERTEX_POINT('',#14957);
#4254=VERTEX_POINT('',#14959);
#4255=VERTEX_POINT('',#14961);
#4256=VERTEX_POINT('',#14965);
#4257=VERTEX_POINT('',#14967);
#4258=VERTEX_POINT('',#14971);
#4259=VERTEX_POINT('',#14972);
#4260=VERTEX_POINT('',#14976);
#4261=VERTEX_POINT('',#14978);
#4262=VERTEX_POINT('',#14984);
#4263=VERTEX_POINT('',#14988);
#4264=VERTEX_POINT('',#14994);
#4265=VERTEX_POINT('',#14995);
#4266=VERTEX_POINT('',#14997);
#4267=VERTEX_POINT('',#14999);
#4268=VERTEX_POINT('',#15003);
#4269=VERTEX_POINT('',#15005);
#4270=VERTEX_POINT('',#15009);
#4271=VERTEX_POINT('',#15010);
#4272=VERTEX_POINT('',#15014);
#4273=VERTEX_POINT('',#15016);
#4274=VERTEX_POINT('',#15022);
#4275=VERTEX_POINT('',#15026);
#4276=VERTEX_POINT('',#15032);
#4277=VERTEX_POINT('',#15033);
#4278=VERTEX_POINT('',#15037);
#4279=VERTEX_POINT('',#15039);
#4280=VERTEX_POINT('',#15045);
#4281=VERTEX_POINT('',#15049);
#4282=VERTEX_POINT('',#15055);
#4283=VERTEX_POINT('',#15057);
#4284=VERTEX_POINT('',#15059);
#4285=VERTEX_POINT('',#15065);
#4286=VERTEX_POINT('',#15067);
#4287=VERTEX_POINT('',#15081);
#4288=VERTEX_POINT('',#15094);
#4289=VERTEX_POINT('',#15106);
#4290=VERTEX_POINT('',#15115);
#4291=VERTEX_POINT('',#15125);
#4292=VERTEX_POINT('',#15132);
#4293=VERTEX_POINT('',#15137);
#4294=VERTEX_POINT('',#15159);
#4295=VERTEX_POINT('',#15163);
#5304=EDGE_CURVE('',#4169,#4170,#2571,.T.);
#5305=EDGE_CURVE('',#4170,#4171,#763,.T.);
#5306=EDGE_CURVE('',#4172,#4171,#2572,.T.);
#5307=EDGE_CURVE('',#4172,#4169,#764,.T.);
#5308=EDGE_CURVE('',#4169,#4173,#2573,.T.);
#5309=EDGE_CURVE('',#4174,#4173,#834,.T.);
#5310=EDGE_CURVE('',#4174,#4170,#2574,.T.);
#5311=EDGE_CURVE('',#4175,#4172,#2575,.T.);
#5312=EDGE_CURVE('',#4176,#4175,#765,.T.);
#5313=EDGE_CURVE('',#4177,#4176,#2576,.T.);
#5314=EDGE_CURVE('',#4177,#4173,#766,.T.);
#5315=EDGE_CURVE('',#4175,#4178,#2577,.T.);
#5316=EDGE_CURVE('',#4178,#4179,#767,.T.);
#5317=EDGE_CURVE('',#4176,#4179,#2578,.T.);
#5318=EDGE_CURVE('',#4171,#4178,#2579,.T.);
#5319=EDGE_CURVE('',#4180,#4181,#2580,.T.);
#5320=EDGE_CURVE('',#4181,#4182,#768,.T.);
#5321=EDGE_CURVE('',#4183,#4182,#2581,.T.);
#5322=EDGE_CURVE('',#4183,#4180,#769,.T.);
#5323=EDGE_CURVE('',#4180,#4184,#2582,.T.);
#5324=EDGE_CURVE('',#4184,#4185,#2583,.T.);
#5325=EDGE_CURVE('',#4185,#4181,#2584,.T.);
#5326=EDGE_CURVE('',#4186,#4183,#2585,.T.);
#5327=EDGE_CURVE('',#4186,#4187,#770,.T.);
#5328=EDGE_CURVE('',#4188,#4187,#2586,.T.);
#5329=EDGE_CURVE('',#4184,#4188,#771,.T.);
#5330=EDGE_CURVE('',#4188,#4189,#2587,.T.);
#5331=EDGE_CURVE('',#4189,#4185,#772,.T.);
#5332=EDGE_CURVE('',#4190,#4187,#835,.T.);
#5333=EDGE_CURVE('',#4190,#4189,#2588,.T.);
#5334=EDGE_CURVE('',#4191,#4192,#2589,.T.);
#5335=EDGE_CURVE('',#4192,#4192,#281,.T.);
#5336=EDGE_CURVE('',#4191,#4191,#282,.T.);
#5337=EDGE_CURVE('',#4192,#4193,#2590,.T.);
#5338=EDGE_CURVE('',#4194,#4193,#283,.T.);
#5339=EDGE_CURVE('',#4193,#4194,#284,.T.);
#5340=EDGE_CURVE('',#4174,#4195,#836,.T.);
#5341=EDGE_CURVE('',#4196,#4177,#837,.F.);
#5342=EDGE_CURVE('',#4197,#4196,#838,.T.);
#5343=EDGE_CURVE('',#4198,#4197,#773,.T.);
#5344=EDGE_CURVE('',#4198,#4199,#2591,.T.);
#5345=EDGE_CURVE('',#4199,#4199,#774,.T.);
#5346=EDGE_CURVE('',#4200,#4198,#775,.T.);
#5347=EDGE_CURVE('',#4190,#4200,#839,.T.);
#5348=EDGE_CURVE('',#4201,#4186,#840,.F.);
#5349=EDGE_CURVE('',#4202,#4201,#841,.T.);
#5350=EDGE_CURVE('',#4195,#4202,#776,.T.);
#5351=EDGE_CURVE('',#4203,#4203,#777,.T.);
#5352=EDGE_CURVE('',#4204,#4205,#119,.T.);
#5353=EDGE_CURVE('',#4206,#4204,#2592,.T.);
#5354=EDGE_CURVE('',#4207,#4206,#120,.T.);
#5355=EDGE_CURVE('',#4205,#4207,#2593,.T.);
#5356=EDGE_CURVE('',#4208,#4204,#121,.T.);
#5357=EDGE_CURVE('',#4209,#4208,#2594,.T.);
#5358=EDGE_CURVE('',#4206,#4209,#122,.T.);
#5359=EDGE_CURVE('',#4210,#4211,#2595,.T.);
#5360=EDGE_CURVE('',#4212,#4210,#2596,.T.);
#5361=EDGE_CURVE('',#4213,#4212,#2597,.T.);
#5362=EDGE_CURVE('',#4211,#4213,#2598,.T.);
#5363=EDGE_CURVE('',#4214,#4210,#2599,.T.);
#5364=EDGE_CURVE('',#4215,#4214,#2600,.T.);
#5365=EDGE_CURVE('',#4212,#4215,#2601,.T.);
#5366=EDGE_CURVE('',#4216,#4217,#2602,.T.);
#5367=EDGE_CURVE('',#4218,#4216,#2603,.T.);
#5368=EDGE_CURVE('',#4219,#4218,#2604,.T.);
#5369=EDGE_CURVE('',#4217,#4219,#2605,.T.);
#5370=EDGE_CURVE('',#4220,#4216,#2606,.T.);
#5371=EDGE_CURVE('',#4221,#4220,#2607,.T.);
#5372=EDGE_CURVE('',#4218,#4221,#2608,.T.);
#5373=EDGE_CURVE('',#4222,#4223,#2609,.T.);
#5374=EDGE_CURVE('',#4224,#4222,#2610,.T.);
#5375=EDGE_CURVE('',#4225,#4224,#2611,.T.);
#5376=EDGE_CURVE('',#4223,#4225,#2612,.T.);
#5377=EDGE_CURVE('',#4226,#4222,#2613,.T.);
#5378=EDGE_CURVE('',#4227,#4226,#2614,.T.);
#5379=EDGE_CURVE('',#4224,#4227,#2615,.T.);
#5380=EDGE_CURVE('',#4228,#4229,#2616,.T.);
#5381=EDGE_CURVE('',#4230,#4228,#2617,.T.);
#5382=EDGE_CURVE('',#4231,#4230,#2618,.T.);
#5383=EDGE_CURVE('',#4229,#4231,#2619,.T.);
#5384=EDGE_CURVE('',#4232,#4228,#2620,.T.);
#5385=EDGE_CURVE('',#4233,#4232,#2621,.T.);
#5386=EDGE_CURVE('',#4230,#4233,#2622,.T.);
#5387=EDGE_CURVE('',#4234,#4235,#123,.T.);
#5388=EDGE_CURVE('',#4234,#4236,#2623,.T.);
#5389=EDGE_CURVE('',#4237,#4236,#124,.T.);
#5390=EDGE_CURVE('',#4235,#4237,#2624,.T.);
#5391=EDGE_CURVE('',#4238,#4234,#125,.T.);
#5392=EDGE_CURVE('',#4239,#4238,#2625,.T.);
#5393=EDGE_CURVE('',#4236,#4239,#126,.T.);
#5394=EDGE_CURVE('',#4240,#4241,#127,.T.);
#5395=EDGE_CURVE('',#4240,#4242,#2626,.T.);
#5396=EDGE_CURVE('',#4243,#4242,#128,.T.);
#5397=EDGE_CURVE('',#4241,#4243,#2627,.T.);
#5398=EDGE_CURVE('',#4244,#4240,#129,.T.);
#5399=EDGE_CURVE('',#4245,#4244,#2628,.T.);
#5400=EDGE_CURVE('',#4242,#4245,#130,.T.);
#5401=EDGE_CURVE('',#4246,#4247,#2629,.T.);
#5402=EDGE_CURVE('',#4248,#4246,#2630,.T.);
#5403=EDGE_CURVE('',#4249,#4248,#2631,.T.);
#5404=EDGE_CURVE('',#4247,#4249,#2632,.T.);
#5405=EDGE_CURVE('',#4250,#4246,#2633,.T.);
#5406=EDGE_CURVE('',#4251,#4250,#2634,.T.);
#5407=EDGE_CURVE('',#4248,#4251,#2635,.T.);
#5408=EDGE_CURVE('',#4252,#4253,#2636,.T.);
#5409=EDGE_CURVE('',#4254,#4252,#2637,.T.);
#5410=EDGE_CURVE('',#4255,#4254,#2638,.T.);
#5411=EDGE_CURVE('',#4253,#4255,#2639,.T.);
#5412=EDGE_CURVE('',#4256,#4252,#2640,.T.);
#5413=EDGE_CURVE('',#4257,#4256,#2641,.T.);
#5414=EDGE_CURVE('',#4254,#4257,#2642,.T.);
#5415=EDGE_CURVE('',#4258,#4259,#131,.T.);
#5416=EDGE_CURVE('',#4258,#4260,#2643,.T.);
#5417=EDGE_CURVE('',#4261,#4260,#132,.T.);
#5418=EDGE_CURVE('',#4259,#4261,#2644,.T.);
#5419=EDGE_CURVE('',#4262,#4258,#133,.T.);
#5420=EDGE_CURVE('',#4263,#4262,#2645,.T.);
#5421=EDGE_CURVE('',#4260,#4263,#134,.T.);
#5422=EDGE_CURVE('',#4264,#4265,#2646,.T.);
#5423=EDGE_CURVE('',#4266,#4264,#2647,.T.);
#5424=EDGE_CURVE('',#4267,#4266,#2648,.T.);
#5425=EDGE_CURVE('',#4265,#4267,#2649,.T.);
#5426=EDGE_CURVE('',#4268,#4264,#2650,.T.);
#5427=EDGE_CURVE('',#4269,#4268,#2651,.T.);
#5428=EDGE_CURVE('',#4266,#4269,#2652,.T.);
#5429=EDGE_CURVE('',#4270,#4271,#135,.T.);
#5430=EDGE_CURVE('',#4272,#4270,#2653,.T.);
#5431=EDGE_CURVE('',#4273,#4272,#136,.T.);
#5432=EDGE_CURVE('',#4271,#4273,#2654,.T.);
#5433=EDGE_CURVE('',#4274,#4270,#137,.T.);
#5434=EDGE_CURVE('',#4275,#4274,#2655,.T.);
#5435=EDGE_CURVE('',#4272,#4275,#138,.T.);
#5436=EDGE_CURVE('',#4276,#4277,#139,.T.);
#5437=EDGE_CURVE('',#4276,#4278,#2656,.T.);
#5438=EDGE_CURVE('',#4279,#4278,#140,.T.);
#5439=EDGE_CURVE('',#4277,#4279,#2657,.T.);
#5440=EDGE_CURVE('',#4280,#4276,#141,.T.);
#5441=EDGE_CURVE('',#4281,#4280,#2658,.T.);
#5442=EDGE_CURVE('',#4278,#4281,#142,.T.);
#5443=EDGE_CURVE('',#4239,#4282,#778,.T.);
#5444=EDGE_CURVE('',#4282,#4283,#2659,.T.);
#5445=EDGE_CURVE('',#4283,#4284,#779,.T.);
#5446=EDGE_CURVE('',#4261,#4284,#2660,.T.);
#5447=EDGE_CURVE('',#4263,#4243,#780,.T.);
#5448=EDGE_CURVE('',#4245,#4237,#781,.T.);
#5449=EDGE_CURVE('',#4211,#4285,#2661,.T.);
#5450=EDGE_CURVE('',#4285,#4286,#2662,.T.);
#5451=EDGE_CURVE('',#4286,#4283,#2663,.T.);
#5452=EDGE_CURVE('',#4282,#4250,#2664,.T.);
#5453=EDGE_CURVE('',#4247,#4232,#2665,.T.);
#5454=EDGE_CURVE('',#4229,#4256,#2666,.T.);
#5455=EDGE_CURVE('',#4253,#4226,#2667,.T.);
#5456=EDGE_CURVE('',#4223,#4220,#2668,.T.);
#5457=EDGE_CURVE('',#4217,#4268,#2669,.T.);
#5458=EDGE_CURVE('',#4265,#4214,#2670,.T.);
#5459=EDGE_CURVE('',#4277,#4207,#782,.T.);
#5460=EDGE_CURVE('',#4205,#4279,#783,.T.);
#5461=EDGE_CURVE('',#4287,#4213,#2671,.T.);
#5462=EDGE_CURVE('',#4275,#4287,#784,.T.);
#5463=EDGE_CURVE('',#4285,#4274,#785,.T.);
#5464=EDGE_CURVE('',#4269,#4219,#2672,.T.);
#5465=EDGE_CURVE('',#4257,#4231,#2673,.T.);
#5466=EDGE_CURVE('',#4241,#4262,#786,.T.);
#5467=EDGE_CURVE('',#4235,#4244,#787,.T.);
#5468=EDGE_CURVE('',#4288,#4238,#788,.T.);
#5469=EDGE_CURVE('',#4251,#4288,#2674,.T.);
#5470=EDGE_CURVE('',#4233,#4249,#2675,.T.);
#5471=EDGE_CURVE('',#4227,#4255,#2676,.T.);
#5472=EDGE_CURVE('',#4221,#4225,#2677,.T.);
#5473=EDGE_CURVE('',#4215,#4267,#2678,.T.);
#5474=EDGE_CURVE('',#4281,#4289,#2679,.T.);
#5475=EDGE_CURVE('',#4289,#4286,#789,.T.);
#5476=EDGE_CURVE('',#4271,#4208,#790,.T.);
#5477=EDGE_CURVE('',#4196,#4190,#2680,.T.);
#5478=EDGE_CURVE('',#4200,#4197,#2681,.T.);
#5479=EDGE_CURVE('',#4179,#4196,#2682,.T.);
#5480=EDGE_CURVE('',#4290,#4179,#2683,.T.);
#5481=EDGE_CURVE('',#4284,#4290,#2684,.T.);
#5482=EDGE_CURVE('',#4189,#4284,#2685,.T.);
#5483=EDGE_CURVE('',#4201,#4174,#2686,.T.);
#5484=EDGE_CURVE('',#4195,#4202,#2687,.T.);
#5485=EDGE_CURVE('',#4182,#4201,#2688,.T.);
#5486=EDGE_CURVE('',#4289,#4182,#2689,.T.);
#5487=EDGE_CURVE('',#4291,#4289,#2690,.T.);
#5488=EDGE_CURVE('',#4170,#4291,#2691,.T.);
#5489=EDGE_CURVE('',#4283,#4185,#2692,.T.);
#5490=EDGE_CURVE('',#4178,#4292,#2693,.T.);
#5491=EDGE_CURVE('',#4290,#4292,#791,.T.);
#5492=EDGE_CURVE('',#4293,#4291,#792,.T.);
#5493=EDGE_CURVE('',#4293,#4171,#2694,.T.);
#5494=EDGE_CURVE('',#4292,#4293,#2695,.T.);
#5495=EDGE_CURVE('',#4259,#4290,#2696,.T.);
#5496=EDGE_CURVE('',#4292,#4288,#2697,.T.);
#5497=EDGE_CURVE('',#4280,#4291,#2698,.T.);
#5498=EDGE_CURVE('',#4209,#4273,#793,.T.);
#5499=EDGE_CURVE('',#4287,#4293,#2699,.T.);
#5500=EDGE_CURVE('',#4181,#4286,#2700,.T.);
#5501=EDGE_CURVE('',#4203,#4294,#2701,.T.);
#5502=EDGE_CURVE('',#4294,#4294,#794,.T.);
#5503=EDGE_CURVE('',#4295,#4295,#795,.T.);
#5504=EDGE_CURVE('',#4199,#4295,#2702,.T.);
#7464=ORIENTED_EDGE('',*,*,#5304,.T.);
#7465=ORIENTED_EDGE('',*,*,#5305,.T.);
#7466=ORIENTED_EDGE('',*,*,#5306,.F.);
#7467=ORIENTED_EDGE('',*,*,#5307,.T.);
#7468=ORIENTED_EDGE('',*,*,#5304,.F.);
#7469=ORIENTED_EDGE('',*,*,#5308,.T.);
#7470=ORIENTED_EDGE('',*,*,#5309,.F.);
#7471=ORIENTED_EDGE('',*,*,#5310,.T.);
#7472=ORIENTED_EDGE('',*,*,#5307,.F.);
#7473=ORIENTED_EDGE('',*,*,#5311,.F.);
#7474=ORIENTED_EDGE('',*,*,#5312,.F.);
#7475=ORIENTED_EDGE('',*,*,#5313,.F.);
#7476=ORIENTED_EDGE('',*,*,#5314,.T.);
#7477=ORIENTED_EDGE('',*,*,#5308,.F.);
#7478=ORIENTED_EDGE('',*,*,#5315,.T.);
#7479=ORIENTED_EDGE('',*,*,#5316,.T.);
#7480=ORIENTED_EDGE('',*,*,#5317,.F.);
#7481=ORIENTED_EDGE('',*,*,#5312,.T.);
#7482=ORIENTED_EDGE('',*,*,#5306,.T.);
#7483=ORIENTED_EDGE('',*,*,#5318,.T.);
#7484=ORIENTED_EDGE('',*,*,#5315,.F.);
#7485=ORIENTED_EDGE('',*,*,#5311,.T.);
#7486=ORIENTED_EDGE('',*,*,#5319,.T.);
#7487=ORIENTED_EDGE('',*,*,#5320,.T.);
#7488=ORIENTED_EDGE('',*,*,#5321,.F.);
#7489=ORIENTED_EDGE('',*,*,#5322,.T.);
#7490=ORIENTED_EDGE('',*,*,#5319,.F.);
#7491=ORIENTED_EDGE('',*,*,#5323,.T.);
#7492=ORIENTED_EDGE('',*,*,#5324,.T.);
#7493=ORIENTED_EDGE('',*,*,#5325,.T.);
#7494=ORIENTED_EDGE('',*,*,#5322,.F.);
#7495=ORIENTED_EDGE('',*,*,#5326,.F.);
#7496=ORIENTED_EDGE('',*,*,#5327,.T.);
#7497=ORIENTED_EDGE('',*,*,#5328,.F.);
#7498=ORIENTED_EDGE('',*,*,#5329,.F.);
#7499=ORIENTED_EDGE('',*,*,#5323,.F.);
#7500=ORIENTED_EDGE('',*,*,#5330,.T.);
#7501=ORIENTED_EDGE('',*,*,#5331,.T.);
#7502=ORIENTED_EDGE('',*,*,#5324,.F.);
#7503=ORIENTED_EDGE('',*,*,#5329,.T.);
#7504=ORIENTED_EDGE('',*,*,#5330,.F.);
#7505=ORIENTED_EDGE('',*,*,#5328,.T.);
#7506=ORIENTED_EDGE('',*,*,#5332,.F.);
#7507=ORIENTED_EDGE('',*,*,#5333,.T.);
#7508=ORIENTED_EDGE('',*,*,#5334,.T.);
#7509=ORIENTED_EDGE('',*,*,#5335,.T.);
#7510=ORIENTED_EDGE('',*,*,#5334,.F.);
#7511=ORIENTED_EDGE('',*,*,#5336,.T.);
#7512=ORIENTED_EDGE('',*,*,#5335,.F.);
#7513=ORIENTED_EDGE('',*,*,#5337,.T.);
#7514=ORIENTED_EDGE('',*,*,#5338,.F.);
#7515=ORIENTED_EDGE('',*,*,#5339,.F.);
#7516=ORIENTED_EDGE('',*,*,#5337,.F.);
#7517=ORIENTED_EDGE('',*,*,#5340,.F.);
#7518=ORIENTED_EDGE('',*,*,#5309,.T.);
#7519=ORIENTED_EDGE('',*,*,#5314,.F.);
#7520=ORIENTED_EDGE('',*,*,#5341,.F.);
#7521=ORIENTED_EDGE('',*,*,#5342,.F.);
#7522=ORIENTED_EDGE('',*,*,#5343,.F.);
#7523=ORIENTED_EDGE('',*,*,#5344,.T.);
#7524=ORIENTED_EDGE('',*,*,#5345,.T.);
#7525=ORIENTED_EDGE('',*,*,#5344,.F.);
#7526=ORIENTED_EDGE('',*,*,#5346,.F.);
#7527=ORIENTED_EDGE('',*,*,#5347,.F.);
#7528=ORIENTED_EDGE('',*,*,#5332,.T.);
#7529=ORIENTED_EDGE('',*,*,#5327,.F.);
#7530=ORIENTED_EDGE('',*,*,#5348,.F.);
#7531=ORIENTED_EDGE('',*,*,#5349,.F.);
#7532=ORIENTED_EDGE('',*,*,#5350,.F.);
#7533=ORIENTED_EDGE('',*,*,#5336,.F.);
#7534=ORIENTED_EDGE('',*,*,#5351,.F.);
#7535=ORIENTED_EDGE('',*,*,#5352,.F.);
#7536=ORIENTED_EDGE('',*,*,#5353,.F.);
#7537=ORIENTED_EDGE('',*,*,#5354,.F.);
#7538=ORIENTED_EDGE('',*,*,#5355,.F.);
#7539=ORIENTED_EDGE('',*,*,#5356,.F.);
#7540=ORIENTED_EDGE('',*,*,#5357,.F.);
#7541=ORIENTED_EDGE('',*,*,#5358,.F.);
#7542=ORIENTED_EDGE('',*,*,#5353,.T.);
#7543=ORIENTED_EDGE('',*,*,#5359,.F.);
#7544=ORIENTED_EDGE('',*,*,#5360,.F.);
#7545=ORIENTED_EDGE('',*,*,#5361,.F.);
#7546=ORIENTED_EDGE('',*,*,#5362,.F.);
#7547=ORIENTED_EDGE('',*,*,#5363,.F.);
#7548=ORIENTED_EDGE('',*,*,#5364,.F.);
#7549=ORIENTED_EDGE('',*,*,#5365,.F.);
#7550=ORIENTED_EDGE('',*,*,#5360,.T.);
#7551=ORIENTED_EDGE('',*,*,#5366,.F.);
#7552=ORIENTED_EDGE('',*,*,#5367,.F.);
#7553=ORIENTED_EDGE('',*,*,#5368,.F.);
#7554=ORIENTED_EDGE('',*,*,#5369,.F.);
#7555=ORIENTED_EDGE('',*,*,#5370,.F.);
#7556=ORIENTED_EDGE('',*,*,#5371,.F.);
#7557=ORIENTED_EDGE('',*,*,#5372,.F.);
#7558=ORIENTED_EDGE('',*,*,#5367,.T.);
#7559=ORIENTED_EDGE('',*,*,#5373,.F.);
#7560=ORIENTED_EDGE('',*,*,#5374,.F.);
#7561=ORIENTED_EDGE('',*,*,#5375,.F.);
#7562=ORIENTED_EDGE('',*,*,#5376,.F.);
#7563=ORIENTED_EDGE('',*,*,#5377,.F.);
#7564=ORIENTED_EDGE('',*,*,#5378,.F.);
#7565=ORIENTED_EDGE('',*,*,#5379,.F.);
#7566=ORIENTED_EDGE('',*,*,#5374,.T.);
#7567=ORIENTED_EDGE('',*,*,#5380,.F.);
#7568=ORIENTED_EDGE('',*,*,#5381,.F.);
#7569=ORIENTED_EDGE('',*,*,#5382,.F.);
#7570=ORIENTED_EDGE('',*,*,#5383,.F.);
#7571=ORIENTED_EDGE('',*,*,#5384,.F.);
#7572=ORIENTED_EDGE('',*,*,#5385,.F.);
#7573=ORIENTED_EDGE('',*,*,#5386,.F.);
#7574=ORIENTED_EDGE('',*,*,#5381,.T.);
#7575=ORIENTED_EDGE('',*,*,#5387,.F.);
#7576=ORIENTED_EDGE('',*,*,#5388,.T.);
#7577=ORIENTED_EDGE('',*,*,#5389,.F.);
#7578=ORIENTED_EDGE('',*,*,#5390,.F.);
#7579=ORIENTED_EDGE('',*,*,#5391,.F.);
#7580=ORIENTED_EDGE('',*,*,#5392,.F.);
#7581=ORIENTED_EDGE('',*,*,#5393,.F.);
#7582=ORIENTED_EDGE('',*,*,#5388,.F.);
#7583=ORIENTED_EDGE('',*,*,#5394,.F.);
#7584=ORIENTED_EDGE('',*,*,#5395,.T.);
#7585=ORIENTED_EDGE('',*,*,#5396,.F.);
#7586=ORIENTED_EDGE('',*,*,#5397,.F.);
#7587=ORIENTED_EDGE('',*,*,#5398,.F.);
#7588=ORIENTED_EDGE('',*,*,#5399,.F.);
#7589=ORIENTED_EDGE('',*,*,#5400,.F.);
#7590=ORIENTED_EDGE('',*,*,#5395,.F.);
#7591=ORIENTED_EDGE('',*,*,#5401,.F.);
#7592=ORIENTED_EDGE('',*,*,#5402,.F.);
#7593=ORIENTED_EDGE('',*,*,#5403,.F.);
#7594=ORIENTED_EDGE('',*,*,#5404,.F.);
#7595=ORIENTED_EDGE('',*,*,#5405,.F.);
#7596=ORIENTED_EDGE('',*,*,#5406,.F.);
#7597=ORIENTED_EDGE('',*,*,#5407,.F.);
#7598=ORIENTED_EDGE('',*,*,#5402,.T.);
#7599=ORIENTED_EDGE('',*,*,#5408,.F.);
#7600=ORIENTED_EDGE('',*,*,#5409,.F.);
#7601=ORIENTED_EDGE('',*,*,#5410,.F.);
#7602=ORIENTED_EDGE('',*,*,#5411,.F.);
#7603=ORIENTED_EDGE('',*,*,#5412,.F.);
#7604=ORIENTED_EDGE('',*,*,#5413,.F.);
#7605=ORIENTED_EDGE('',*,*,#5414,.F.);
#7606=ORIENTED_EDGE('',*,*,#5409,.T.);
#7607=ORIENTED_EDGE('',*,*,#5415,.F.);
#7608=ORIENTED_EDGE('',*,*,#5416,.T.);
#7609=ORIENTED_EDGE('',*,*,#5417,.F.);
#7610=ORIENTED_EDGE('',*,*,#5418,.F.);
#7611=ORIENTED_EDGE('',*,*,#5419,.F.);
#7612=ORIENTED_EDGE('',*,*,#5420,.F.);
#7613=ORIENTED_EDGE('',*,*,#5421,.F.);
#7614=ORIENTED_EDGE('',*,*,#5416,.F.);
#7615=ORIENTED_EDGE('',*,*,#5422,.F.);
#7616=ORIENTED_EDGE('',*,*,#5423,.F.);
#7617=ORIENTED_EDGE('',*,*,#5424,.F.);
#7618=ORIENTED_EDGE('',*,*,#5425,.F.);
#7619=ORIENTED_EDGE('',*,*,#5426,.F.);
#7620=ORIENTED_EDGE('',*,*,#5427,.F.);
#7621=ORIENTED_EDGE('',*,*,#5428,.F.);
#7622=ORIENTED_EDGE('',*,*,#5423,.T.);
#7623=ORIENTED_EDGE('',*,*,#5429,.F.);
#7624=ORIENTED_EDGE('',*,*,#5430,.F.);
#7625=ORIENTED_EDGE('',*,*,#5431,.F.);
#7626=ORIENTED_EDGE('',*,*,#5432,.F.);
#7627=ORIENTED_EDGE('',*,*,#5433,.F.);
#7628=ORIENTED_EDGE('',*,*,#5434,.F.);
#7629=ORIENTED_EDGE('',*,*,#5435,.F.);
#7630=ORIENTED_EDGE('',*,*,#5430,.T.);
#7631=ORIENTED_EDGE('',*,*,#5436,.F.);
#7632=ORIENTED_EDGE('',*,*,#5437,.T.);
#7633=ORIENTED_EDGE('',*,*,#5438,.F.);
#7634=ORIENTED_EDGE('',*,*,#5439,.F.);
#7635=ORIENTED_EDGE('',*,*,#5440,.F.);
#7636=ORIENTED_EDGE('',*,*,#5441,.F.);
#7637=ORIENTED_EDGE('',*,*,#5442,.F.);
#7638=ORIENTED_EDGE('',*,*,#5437,.F.);
#7639=ORIENTED_EDGE('',*,*,#5389,.T.);
#7640=ORIENTED_EDGE('',*,*,#5393,.T.);
#7641=ORIENTED_EDGE('',*,*,#5443,.T.);
#7642=ORIENTED_EDGE('',*,*,#5444,.T.);
#7643=ORIENTED_EDGE('',*,*,#5445,.T.);
#7644=ORIENTED_EDGE('',*,*,#5446,.F.);
#7645=ORIENTED_EDGE('',*,*,#5417,.T.);
#7646=ORIENTED_EDGE('',*,*,#5421,.T.);
#7647=ORIENTED_EDGE('',*,*,#5447,.T.);
#7648=ORIENTED_EDGE('',*,*,#5396,.T.);
#7649=ORIENTED_EDGE('',*,*,#5400,.T.);
#7650=ORIENTED_EDGE('',*,*,#5448,.T.);
#7651=ORIENTED_EDGE('',*,*,#5363,.T.);
#7652=ORIENTED_EDGE('',*,*,#5359,.T.);
#7653=ORIENTED_EDGE('',*,*,#5449,.T.);
#7654=ORIENTED_EDGE('',*,*,#5450,.T.);
#7655=ORIENTED_EDGE('',*,*,#5451,.T.);
#7656=ORIENTED_EDGE('',*,*,#5444,.F.);
#7657=ORIENTED_EDGE('',*,*,#5452,.T.);
#7658=ORIENTED_EDGE('',*,*,#5405,.T.);
#7659=ORIENTED_EDGE('',*,*,#5401,.T.);
#7660=ORIENTED_EDGE('',*,*,#5453,.T.);
#7661=ORIENTED_EDGE('',*,*,#5384,.T.);
#7662=ORIENTED_EDGE('',*,*,#5380,.T.);
#7663=ORIENTED_EDGE('',*,*,#5454,.T.);
#7664=ORIENTED_EDGE('',*,*,#5412,.T.);
#7665=ORIENTED_EDGE('',*,*,#5408,.T.);
#7666=ORIENTED_EDGE('',*,*,#5455,.T.);
#7667=ORIENTED_EDGE('',*,*,#5377,.T.);
#7668=ORIENTED_EDGE('',*,*,#5373,.T.);
#7669=ORIENTED_EDGE('',*,*,#5456,.T.);
#7670=ORIENTED_EDGE('',*,*,#5370,.T.);
#7671=ORIENTED_EDGE('',*,*,#5366,.T.);
#7672=ORIENTED_EDGE('',*,*,#5457,.T.);
#7673=ORIENTED_EDGE('',*,*,#5426,.T.);
#7674=ORIENTED_EDGE('',*,*,#5422,.T.);
#7675=ORIENTED_EDGE('',*,*,#5458,.T.);
#7676=ORIENTED_EDGE('',*,*,#5355,.T.);
#7677=ORIENTED_EDGE('',*,*,#5459,.F.);
#7678=ORIENTED_EDGE('',*,*,#5439,.T.);
#7679=ORIENTED_EDGE('',*,*,#5460,.F.);
#7680=ORIENTED_EDGE('',*,*,#5362,.T.);
#7681=ORIENTED_EDGE('',*,*,#5461,.F.);
#7682=ORIENTED_EDGE('',*,*,#5462,.F.);
#7683=ORIENTED_EDGE('',*,*,#5434,.T.);
#7684=ORIENTED_EDGE('',*,*,#5463,.F.);
#7685=ORIENTED_EDGE('',*,*,#5449,.F.);
#7686=ORIENTED_EDGE('',*,*,#5369,.T.);
#7687=ORIENTED_EDGE('',*,*,#5464,.F.);
#7688=ORIENTED_EDGE('',*,*,#5427,.T.);
#7689=ORIENTED_EDGE('',*,*,#5457,.F.);
#7690=ORIENTED_EDGE('',*,*,#5383,.T.);
#7691=ORIENTED_EDGE('',*,*,#5465,.F.);
#7692=ORIENTED_EDGE('',*,*,#5413,.T.);
#7693=ORIENTED_EDGE('',*,*,#5454,.F.);
#7694=ORIENTED_EDGE('',*,*,#5397,.T.);
#7695=ORIENTED_EDGE('',*,*,#5447,.F.);
#7696=ORIENTED_EDGE('',*,*,#5420,.T.);
#7697=ORIENTED_EDGE('',*,*,#5466,.F.);
#7698=ORIENTED_EDGE('',*,*,#5390,.T.);
#7699=ORIENTED_EDGE('',*,*,#5448,.F.);
#7700=ORIENTED_EDGE('',*,*,#5399,.T.);
#7701=ORIENTED_EDGE('',*,*,#5467,.F.);
#7702=ORIENTED_EDGE('',*,*,#5392,.T.);
#7703=ORIENTED_EDGE('',*,*,#5468,.F.);
#7704=ORIENTED_EDGE('',*,*,#5469,.F.);
#7705=ORIENTED_EDGE('',*,*,#5406,.T.);
#7706=ORIENTED_EDGE('',*,*,#5452,.F.);
#7707=ORIENTED_EDGE('',*,*,#5443,.F.);
#7708=ORIENTED_EDGE('',*,*,#5385,.T.);
#7709=ORIENTED_EDGE('',*,*,#5453,.F.);
#7710=ORIENTED_EDGE('',*,*,#5404,.T.);
#7711=ORIENTED_EDGE('',*,*,#5470,.F.);
#7712=ORIENTED_EDGE('',*,*,#5378,.T.);
#7713=ORIENTED_EDGE('',*,*,#5455,.F.);
#7714=ORIENTED_EDGE('',*,*,#5411,.T.);
#7715=ORIENTED_EDGE('',*,*,#5471,.F.);
#7716=ORIENTED_EDGE('',*,*,#5371,.T.);
#7717=ORIENTED_EDGE('',*,*,#5456,.F.);
#7718=ORIENTED_EDGE('',*,*,#5376,.T.);
#7719=ORIENTED_EDGE('',*,*,#5472,.F.);
#7720=ORIENTED_EDGE('',*,*,#5364,.T.);
#7721=ORIENTED_EDGE('',*,*,#5458,.F.);
#7722=ORIENTED_EDGE('',*,*,#5425,.T.);
#7723=ORIENTED_EDGE('',*,*,#5473,.F.);
#7724=ORIENTED_EDGE('',*,*,#5356,.T.);
#7725=ORIENTED_EDGE('',*,*,#5352,.T.);
#7726=ORIENTED_EDGE('',*,*,#5460,.T.);
#7727=ORIENTED_EDGE('',*,*,#5438,.T.);
#7728=ORIENTED_EDGE('',*,*,#5442,.T.);
#7729=ORIENTED_EDGE('',*,*,#5474,.T.);
#7730=ORIENTED_EDGE('',*,*,#5475,.T.);
#7731=ORIENTED_EDGE('',*,*,#5450,.F.);
#7732=ORIENTED_EDGE('',*,*,#5463,.T.);
#7733=ORIENTED_EDGE('',*,*,#5433,.T.);
#7734=ORIENTED_EDGE('',*,*,#5429,.T.);
#7735=ORIENTED_EDGE('',*,*,#5476,.T.);
#7736=ORIENTED_EDGE('',*,*,#5342,.T.);
#7737=ORIENTED_EDGE('',*,*,#5477,.T.);
#7738=ORIENTED_EDGE('',*,*,#5347,.T.);
#7739=ORIENTED_EDGE('',*,*,#5478,.T.);
#7740=ORIENTED_EDGE('',*,*,#5477,.F.);
#7741=ORIENTED_EDGE('',*,*,#5479,.F.);
#7742=ORIENTED_EDGE('',*,*,#5480,.F.);
#7743=ORIENTED_EDGE('',*,*,#5481,.F.);
#7744=ORIENTED_EDGE('',*,*,#5482,.F.);
#7745=ORIENTED_EDGE('',*,*,#5333,.F.);
#7746=ORIENTED_EDGE('',*,*,#5349,.T.);
#7747=ORIENTED_EDGE('',*,*,#5483,.T.);
#7748=ORIENTED_EDGE('',*,*,#5340,.T.);
#7749=ORIENTED_EDGE('',*,*,#5484,.T.);
#7750=ORIENTED_EDGE('',*,*,#5483,.F.);
#7751=ORIENTED_EDGE('',*,*,#5485,.F.);
#7752=ORIENTED_EDGE('',*,*,#5486,.F.);
#7753=ORIENTED_EDGE('',*,*,#5487,.F.);
#7754=ORIENTED_EDGE('',*,*,#5488,.F.);
#7755=ORIENTED_EDGE('',*,*,#5310,.F.);
#7756=ORIENTED_EDGE('',*,*,#5331,.F.);
#7757=ORIENTED_EDGE('',*,*,#5482,.T.);
#7758=ORIENTED_EDGE('',*,*,#5445,.F.);
#7759=ORIENTED_EDGE('',*,*,#5489,.T.);
#7760=ORIENTED_EDGE('',*,*,#5317,.T.);
#7761=ORIENTED_EDGE('',*,*,#5479,.T.);
#7762=ORIENTED_EDGE('',*,*,#5341,.T.);
#7763=ORIENTED_EDGE('',*,*,#5313,.T.);
#7764=ORIENTED_EDGE('',*,*,#5316,.F.);
#7765=ORIENTED_EDGE('',*,*,#5490,.T.);
#7766=ORIENTED_EDGE('',*,*,#5491,.F.);
#7767=ORIENTED_EDGE('',*,*,#5480,.T.);
#7768=ORIENTED_EDGE('',*,*,#5321,.T.);
#7769=ORIENTED_EDGE('',*,*,#5485,.T.);
#7770=ORIENTED_EDGE('',*,*,#5348,.T.);
#7771=ORIENTED_EDGE('',*,*,#5326,.T.);
#7772=ORIENTED_EDGE('',*,*,#5305,.F.);
#7773=ORIENTED_EDGE('',*,*,#5488,.T.);
#7774=ORIENTED_EDGE('',*,*,#5492,.F.);
#7775=ORIENTED_EDGE('',*,*,#5493,.T.);
#7776=ORIENTED_EDGE('',*,*,#5318,.F.);
#7777=ORIENTED_EDGE('',*,*,#5493,.F.);
#7778=ORIENTED_EDGE('',*,*,#5494,.F.);
#7779=ORIENTED_EDGE('',*,*,#5490,.F.);
#7780=ORIENTED_EDGE('',*,*,#5387,.T.);
#7781=ORIENTED_EDGE('',*,*,#5467,.T.);
#7782=ORIENTED_EDGE('',*,*,#5398,.T.);
#7783=ORIENTED_EDGE('',*,*,#5394,.T.);
#7784=ORIENTED_EDGE('',*,*,#5466,.T.);
#7785=ORIENTED_EDGE('',*,*,#5419,.T.);
#7786=ORIENTED_EDGE('',*,*,#5415,.T.);
#7787=ORIENTED_EDGE('',*,*,#5495,.T.);
#7788=ORIENTED_EDGE('',*,*,#5491,.T.);
#7789=ORIENTED_EDGE('',*,*,#5496,.T.);
#7790=ORIENTED_EDGE('',*,*,#5468,.T.);
#7791=ORIENTED_EDGE('',*,*,#5391,.T.);
#7792=ORIENTED_EDGE('',*,*,#5495,.F.);
#7793=ORIENTED_EDGE('',*,*,#5418,.T.);
#7794=ORIENTED_EDGE('',*,*,#5446,.T.);
#7795=ORIENTED_EDGE('',*,*,#5481,.T.);
#7796=ORIENTED_EDGE('',*,*,#5474,.F.);
#7797=ORIENTED_EDGE('',*,*,#5441,.T.);
#7798=ORIENTED_EDGE('',*,*,#5497,.T.);
#7799=ORIENTED_EDGE('',*,*,#5487,.T.);
#7800=ORIENTED_EDGE('',*,*,#5358,.T.);
#7801=ORIENTED_EDGE('',*,*,#5498,.T.);
#7802=ORIENTED_EDGE('',*,*,#5431,.T.);
#7803=ORIENTED_EDGE('',*,*,#5435,.T.);
#7804=ORIENTED_EDGE('',*,*,#5462,.T.);
#7805=ORIENTED_EDGE('',*,*,#5499,.T.);
#7806=ORIENTED_EDGE('',*,*,#5492,.T.);
#7807=ORIENTED_EDGE('',*,*,#5497,.F.);
#7808=ORIENTED_EDGE('',*,*,#5440,.T.);
#7809=ORIENTED_EDGE('',*,*,#5436,.T.);
#7810=ORIENTED_EDGE('',*,*,#5459,.T.);
#7811=ORIENTED_EDGE('',*,*,#5354,.T.);
#7812=ORIENTED_EDGE('',*,*,#5365,.T.);
#7813=ORIENTED_EDGE('',*,*,#5473,.T.);
#7814=ORIENTED_EDGE('',*,*,#5424,.T.);
#7815=ORIENTED_EDGE('',*,*,#5428,.T.);
#7816=ORIENTED_EDGE('',*,*,#5464,.T.);
#7817=ORIENTED_EDGE('',*,*,#5368,.T.);
#7818=ORIENTED_EDGE('',*,*,#5372,.T.);
#7819=ORIENTED_EDGE('',*,*,#5472,.T.);
#7820=ORIENTED_EDGE('',*,*,#5375,.T.);
#7821=ORIENTED_EDGE('',*,*,#5379,.T.);
#7822=ORIENTED_EDGE('',*,*,#5471,.T.);
#7823=ORIENTED_EDGE('',*,*,#5410,.T.);
#7824=ORIENTED_EDGE('',*,*,#5414,.T.);
#7825=ORIENTED_EDGE('',*,*,#5465,.T.);
#7826=ORIENTED_EDGE('',*,*,#5382,.T.);
#7827=ORIENTED_EDGE('',*,*,#5386,.T.);
#7828=ORIENTED_EDGE('',*,*,#5470,.T.);
#7829=ORIENTED_EDGE('',*,*,#5403,.T.);
#7830=ORIENTED_EDGE('',*,*,#5407,.T.);
#7831=ORIENTED_EDGE('',*,*,#5469,.T.);
#7832=ORIENTED_EDGE('',*,*,#5496,.F.);
#7833=ORIENTED_EDGE('',*,*,#5494,.T.);
#7834=ORIENTED_EDGE('',*,*,#5499,.F.);
#7835=ORIENTED_EDGE('',*,*,#5461,.T.);
#7836=ORIENTED_EDGE('',*,*,#5361,.T.);
#7837=ORIENTED_EDGE('',*,*,#5357,.T.);
#7838=ORIENTED_EDGE('',*,*,#5476,.F.);
#7839=ORIENTED_EDGE('',*,*,#5432,.T.);
#7840=ORIENTED_EDGE('',*,*,#5498,.F.);
#7841=ORIENTED_EDGE('',*,*,#5320,.F.);
#7842=ORIENTED_EDGE('',*,*,#5500,.T.);
#7843=ORIENTED_EDGE('',*,*,#5475,.F.);
#7844=ORIENTED_EDGE('',*,*,#5486,.T.);
#7845=ORIENTED_EDGE('',*,*,#5325,.F.);
#7846=ORIENTED_EDGE('',*,*,#5489,.F.);
#7847=ORIENTED_EDGE('',*,*,#5451,.F.);
#7848=ORIENTED_EDGE('',*,*,#5500,.F.);
#7849=ORIENTED_EDGE('',*,*,#5478,.F.);
#7850=ORIENTED_EDGE('',*,*,#5346,.T.);
#7851=ORIENTED_EDGE('',*,*,#5343,.T.);
#7852=ORIENTED_EDGE('',*,*,#5484,.F.);
#7853=ORIENTED_EDGE('',*,*,#5350,.T.);
#7854=ORIENTED_EDGE('',*,*,#5351,.T.);
#7855=ORIENTED_EDGE('',*,*,#5501,.T.);
#7856=ORIENTED_EDGE('',*,*,#5502,.F.);
#7857=ORIENTED_EDGE('',*,*,#5501,.F.);
#7858=ORIENTED_EDGE('',*,*,#5338,.T.);
#7859=ORIENTED_EDGE('',*,*,#5339,.T.);
#7860=ORIENTED_EDGE('',*,*,#5503,.F.);
#7861=ORIENTED_EDGE('',*,*,#5502,.T.);
#7862=ORIENTED_EDGE('',*,*,#5345,.F.);
#7863=ORIENTED_EDGE('',*,*,#5504,.T.);
#7864=ORIENTED_EDGE('',*,*,#5503,.T.);
#7865=ORIENTED_EDGE('',*,*,#5504,.F.);
#8479=PLANE('',#9733);
#8480=PLANE('',#9735);
#8481=PLANE('',#9740);
#8482=PLANE('',#9744);
#8483=PLANE('',#9745);
#8484=PLANE('',#9750);
#8485=PLANE('',#9764);
#8486=PLANE('',#9766);
#8487=PLANE('',#9767);
#8488=PLANE('',#9768);
#8489=PLANE('',#9769);
#8490=PLANE('',#9770);
#8491=PLANE('',#9771);
#8492=PLANE('',#9772);
#8493=PLANE('',#9773);
#8494=PLANE('',#9774);
#8495=PLANE('',#9775);
#8496=PLANE('',#9776);
#8497=PLANE('',#9777);
#8498=PLANE('',#9778);
#8499=PLANE('',#9779);
#8500=PLANE('',#9780);
#8501=PLANE('',#9781);
#8502=PLANE('',#9782);
#8503=PLANE('',#9783);
#8504=PLANE('',#9784);
#8505=PLANE('',#9785);
#8506=PLANE('',#9786);
#8507=PLANE('',#9787);
#8508=PLANE('',#9788);
#8509=PLANE('',#9789);
#8510=PLANE('',#9790);
#8511=PLANE('',#9791);
#8512=PLANE('',#9797);
#8513=PLANE('',#9798);
#8514=PLANE('',#9801);
#8515=PLANE('',#9804);
#8516=PLANE('',#9805);
#8517=PLANE('',#9806);
#8518=PLANE('',#9808);
#8519=PLANE('',#9810);
#8520=PLANE('',#9812);
#8521=PLANE('',#9813);
#8522=PLANE('',#9814);
#8523=PLANE('',#9815);
#8524=PLANE('',#9819);
#8525=PLANE('',#9820);
#8526=PLANE('',#9821);
#8527=PLANE('',#9822);
#8528=PLANE('',#9824);
#8529=PLANE('',#9827);
#8530=PLANE('',#9830);
#8531=PLANE('',#9832);
#8532=PLANE('',#9833);
#8533=PLANE('',#9836);
#8534=PLANE('',#9837);
#8535=PLANE('',#9839);
#8536=PLANE('',#9840);
#8537=PLANE('',#9841);
#8538=PLANE('',#9844);
#8934=ADVANCED_FACE('',(#1213),#421,.T.);
#8935=ADVANCED_FACE('',(#1214),#8479,.T.);
#8936=ADVANCED_FACE('',(#1215),#8480,.F.);
#8937=ADVANCED_FACE('',(#1216),#422,.T.);
#8938=ADVANCED_FACE('',(#1217),#8481,.T.);
#8939=ADVANCED_FACE('',(#1218),#423,.T.);
#8940=ADVANCED_FACE('',(#1219),#8482,.T.);
#8941=ADVANCED_FACE('',(#1220),#8483,.F.);
#8942=ADVANCED_FACE('',(#1221),#424,.T.);
#8943=ADVANCED_FACE('',(#1222),#8484,.T.);
#8944=ADVANCED_FACE('',(#1223),#183,.T.);
#8945=ADVANCED_FACE('',(#1224),#533,.F.);
#8946=ADVANCED_FACE('',(#1225,#623),#534,.T.);
#8947=ADVANCED_FACE('',(#1226),#8485,.F.);
#8948=ADVANCED_FACE('',(#1227),#8486,.F.);
#8949=ADVANCED_FACE('',(#1228),#8487,.F.);
#8950=ADVANCED_FACE('',(#1229),#8488,.F.);
#8951=ADVANCED_FACE('',(#1230),#8489,.F.);
#8952=ADVANCED_FACE('',(#1231),#8490,.F.);
#8953=ADVANCED_FACE('',(#1232),#8491,.F.);
#8954=ADVANCED_FACE('',(#1233),#8492,.F.);
#8955=ADVANCED_FACE('',(#1234),#8493,.F.);
#8956=ADVANCED_FACE('',(#1235),#8494,.F.);
#8957=ADVANCED_FACE('',(#1236),#8495,.F.);
#8958=ADVANCED_FACE('',(#1237),#8496,.F.);
#8959=ADVANCED_FACE('',(#1238),#8497,.F.);
#8960=ADVANCED_FACE('',(#1239),#8498,.F.);
#8961=ADVANCED_FACE('',(#1240),#8499,.F.);
#8962=ADVANCED_FACE('',(#1241),#8500,.F.);
#8963=ADVANCED_FACE('',(#1242),#8501,.F.);
#8964=ADVANCED_FACE('',(#1243),#8502,.F.);
#8965=ADVANCED_FACE('',(#1244),#8503,.F.);
#8966=ADVANCED_FACE('',(#1245),#8504,.F.);
#8967=ADVANCED_FACE('',(#1246),#8505,.F.);
#8968=ADVANCED_FACE('',(#1247),#8506,.F.);
#8969=ADVANCED_FACE('',(#1248),#8507,.F.);
#8970=ADVANCED_FACE('',(#1249),#8508,.F.);
#8971=ADVANCED_FACE('',(#1250),#8509,.F.);
#8972=ADVANCED_FACE('',(#1251),#8510,.F.);
#8973=ADVANCED_FACE('',(#1252),#8511,.F.);
#8974=ADVANCED_FACE('',(#1253),#425,.T.);
#8975=ADVANCED_FACE('',(#1254),#8512,.T.);
#8976=ADVANCED_FACE('',(#1255),#8513,.T.);
#8977=ADVANCED_FACE('',(#1256),#8514,.T.);
#8978=ADVANCED_FACE('',(#1257),#8515,.T.);
#8979=ADVANCED_FACE('',(#1258),#8516,.T.);
#8980=ADVANCED_FACE('',(#1259),#8517,.T.);
#8981=ADVANCED_FACE('',(#1260),#8518,.T.);
#8982=ADVANCED_FACE('',(#1261),#8519,.T.);
#8983=ADVANCED_FACE('',(#1262),#8520,.T.);
#8984=ADVANCED_FACE('',(#1263),#8521,.T.);
#8985=ADVANCED_FACE('',(#1264),#8522,.T.);
#8986=ADVANCED_FACE('',(#1265),#8523,.T.);
#8987=ADVANCED_FACE('',(#1266),#426,.T.);
#8988=ADVANCED_FACE('',(#1267),#8524,.T.);
#8989=ADVANCED_FACE('',(#1268),#8525,.T.);
#8990=ADVANCED_FACE('',(#1269),#8526,.T.);
#8991=ADVANCED_FACE('',(#1270),#8527,.T.);
#8992=ADVANCED_FACE('',(#1271),#535,.T.);
#8993=ADVANCED_FACE('',(#1272),#8528,.T.);
#8994=ADVANCED_FACE('',(#1273),#536,.T.);
#8995=ADVANCED_FACE('',(#1274),#8529,.T.);
#8996=ADVANCED_FACE('',(#1275),#537,.T.);
#8997=ADVANCED_FACE('',(#1276),#8530,.T.);
#8998=ADVANCED_FACE('',(#1277),#427,.T.);
#8999=ADVANCED_FACE('',(#1278),#8531,.T.);
#9000=ADVANCED_FACE('',(#1279),#8532,.T.);
#9001=ADVANCED_FACE('',(#1280),#428,.T.);
#9002=ADVANCED_FACE('',(#1281),#8533,.T.);
#9003=ADVANCED_FACE('',(#1282),#8534,.T.);
#9004=ADVANCED_FACE('',(#1283),#538,.T.);
#9005=ADVANCED_FACE('',(#1284),#8535,.T.);
#9006=ADVANCED_FACE('',(#1285),#8536,.T.);
#9007=ADVANCED_FACE('',(#1286),#8537,.T.);
#9008=ADVANCED_FACE('',(#1287,#624),#539,.F.);
#9009=ADVANCED_FACE('',(#1288,#625),#8538,.T.);
#9010=ADVANCED_FACE('',(#1289),#429,.T.);
#9094=CLOSED_SHELL('',(#8934,#8935,#8936,#8937,#8938,#8939,#8940,#8941,
#8942,#8943,#8944,#8945,#8946,#8947,#8948,#8949,#8950,#8951,#8952,#8953,
#8954,#8955,#8956,#8957,#8958,#8959,#8960,#8961,#8962,#8963,#8964,#8965,
#8966,#8967,#8968,#8969,#8970,#8971,#8972,#8973,#8974,#8975,#8976,#8977,
#8978,#8979,#8980,#8981,#8982,#8983,#8984,#8985,#8986,#8987,#8988,#8989,
#8990,#8991,#8992,#8993,#8994,#8995,#8996,#8997,#8998,#8999,#9000,#9001,
#9002,#9003,#9004,#9005,#9006,#9007,#9008,#9009,#9010));
#9729=AXIS2_PLACEMENT_3D('',#14562,#11579,#11580);
#9730=AXIS2_PLACEMENT_3D('',#14563,#11581,#11582);
#9731=AXIS2_PLACEMENT_3D('',#14568,#11584,#11585);
#9732=AXIS2_PLACEMENT_3D('',#14571,#11587,#11588);
#9733=AXIS2_PLACEMENT_3D('',#14572,#11589,#11590);
#9734=AXIS2_PLACEMENT_3D('',#14576,#11592,#11593);
#9735=AXIS2_PLACEMENT_3D('',#14578,#11595,#11596);
#9736=AXIS2_PLACEMENT_3D('',#14582,#11598,#11599);
#9737=AXIS2_PLACEMENT_3D('',#14585,#11601,#11602);
#9738=AXIS2_PLACEMENT_3D('',#14586,#11603,#11604);
#9739=AXIS2_PLACEMENT_3D('',#14590,#11606,#11607);
#9740=AXIS2_PLACEMENT_3D('',#14592,#11609,#11610);
#9741=AXIS2_PLACEMENT_3D('',#14594,#11612,#11613);
#9742=AXIS2_PLACEMENT_3D('',#14599,#11615,#11616);
#9743=AXIS2_PLACEMENT_3D('',#14602,#11618,#11619);
#9744=AXIS2_PLACEMENT_3D('',#14603,#11620,#11621);
#9745=AXIS2_PLACEMENT_3D('',#14609,#11625,#11626);
#9746=AXIS2_PLACEMENT_3D('',#14613,#11628,#11629);
#9747=AXIS2_PLACEMENT_3D('',#14616,#11631,#11632);
#9748=AXIS2_PLACEMENT_3D('',#14617,#11633,#11634);
#9749=AXIS2_PLACEMENT_3D('',#14620,#11636,#11637);
#9750=AXIS2_PLACEMENT_3D('',#14621,#11638,#11639);
#9751=AXIS2_PLACEMENT_3D('',#14623,#11640,#11641);
#9752=AXIS2_PLACEMENT_3D('',#14748,#11644,#11645);
#9753=AXIS2_PLACEMENT_3D('',#14788,#11647,#11648);
#9754=AXIS2_PLACEMENT_3D('',#14790,#11649,#11650);
#9755=AXIS2_PLACEMENT_3D('',#14792,#11651,#11652);
#9756=AXIS2_PLACEMENT_3D('',#14794,#11653,#11654);
#9757=AXIS2_PLACEMENT_3D('',#14796,#11655,#11656);
#9758=AXIS2_PLACEMENT_3D('',#14799,#11658,#11659);
#9759=AXIS2_PLACEMENT_3D('',#14801,#11660,#11661);
#9760=AXIS2_PLACEMENT_3D('',#14802,#11662,#11663);
#9761=AXIS2_PLACEMENT_3D('',#14804,#11664,#11665);
#9762=AXIS2_PLACEMENT_3D('',#14806,#11666,#11667);
#9763=AXIS2_PLACEMENT_3D('',#14807,#11668,#11669);
#9764=AXIS2_PLACEMENT_3D('',#14808,#11670,#11671);
#9765=AXIS2_PLACEMENT_3D('',#14810,#11672,#11673);
#9766=AXIS2_PLACEMENT_3D('',#14811,#11674,#11675);
#9767=AXIS2_PLACEMENT_3D('',#14824,#11678,#11679);
#9768=AXIS2_PLACEMENT_3D('',#14834,#11681,#11682);
#9769=AXIS2_PLACEMENT_3D('',#14843,#11687,#11688);
#9770=AXIS2_PLACEMENT_3D('',#14849,#11692,#11693);
#9771=AXIS2_PLACEMENT_3D('',#14858,#11698,#11699);
#9772=AXIS2_PLACEMENT_3D('',#14864,#11703,#11704);
#9773=AXIS2_PLACEMENT_3D('',#14873,#11709,#11710);
#9774=AXIS2_PLACEMENT_3D('',#14879,#11714,#11715);
#9775=AXIS2_PLACEMENT_3D('',#14888,#11720,#11721);
#9776=AXIS2_PLACEMENT_3D('',#14894,#11725,#11726);
#9777=AXIS2_PLACEMENT_3D('',#14907,#11729,#11730);
#9778=AXIS2_PLACEMENT_3D('',#14917,#11732,#11733);
#9779=AXIS2_PLACEMENT_3D('',#14930,#11736,#11737);
#9780=AXIS2_PLACEMENT_3D('',#14940,#11739,#11740);
#9781=AXIS2_PLACEMENT_3D('',#14949,#11745,#11746);
#9782=AXIS2_PLACEMENT_3D('',#14955,#11750,#11751);
#9783=AXIS2_PLACEMENT_3D('',#14964,#11756,#11757);
#9784=AXIS2_PLACEMENT_3D('',#14970,#11761,#11762);
#9785=AXIS2_PLACEMENT_3D('',#14983,#11765,#11766);
#9786=AXIS2_PLACEMENT_3D('',#14993,#11768,#11769);
#9787=AXIS2_PLACEMENT_3D('',#15002,#11774,#11775);
#9788=AXIS2_PLACEMENT_3D('',#15008,#11779,#11780);
#9789=AXIS2_PLACEMENT_3D('',#15021,#11783,#11784);
#9790=AXIS2_PLACEMENT_3D('',#15031,#11786,#11787);
#9791=AXIS2_PLACEMENT_3D('',#15044,#11790,#11791);
#9792=AXIS2_PLACEMENT_3D('',#15054,#11793,#11794);
#9793=AXIS2_PLACEMENT_3D('',#15056,#11795,#11796);
#9794=AXIS2_PLACEMENT_3D('',#15060,#11798,#11799);
#9795=AXIS2_PLACEMENT_3D('',#15062,#11801,#11802);
#9796=AXIS2_PLACEMENT_3D('',#15063,#11803,#11804);
#9797=AXIS2_PLACEMENT_3D('',#15064,#11805,#11806);
#9798=AXIS2_PLACEMENT_3D('',#15077,#11817,#11818);
#9799=AXIS2_PLACEMENT_3D('',#15078,#11819,#11820);
#9800=AXIS2_PLACEMENT_3D('',#15079,#11821,#11822);
#9801=AXIS2_PLACEMENT_3D('',#15080,#11823,#11824);
#9802=AXIS2_PLACEMENT_3D('',#15083,#11826,#11827);
#9803=AXIS2_PLACEMENT_3D('',#15084,#11828,#11829);
#9804=AXIS2_PLACEMENT_3D('',#15085,#11830,#11831);
#9805=AXIS2_PLACEMENT_3D('',#15087,#11833,#11834);
#9806=AXIS2_PLACEMENT_3D('',#15089,#11836,#11837);
#9807=AXIS2_PLACEMENT_3D('',#15090,#11838,#11839);
#9808=AXIS2_PLACEMENT_3D('',#15091,#11840,#11841);
#9809=AXIS2_PLACEMENT_3D('',#15092,#11842,#11843);
#9810=AXIS2_PLACEMENT_3D('',#15093,#11844,#11845);
#9811=AXIS2_PLACEMENT_3D('',#15095,#11846,#11847);
#9812=AXIS2_PLACEMENT_3D('',#15097,#11849,#11850);
#9813=AXIS2_PLACEMENT_3D('',#15099,#11852,#11853);
#9814=AXIS2_PLACEMENT_3D('',#15101,#11855,#11856);
#9815=AXIS2_PLACEMENT_3D('',#15103,#11858,#11859);
#9816=AXIS2_PLACEMENT_3D('',#15105,#11861,#11862);
#9817=AXIS2_PLACEMENT_3D('',#15108,#11864,#11865);
#9818=AXIS2_PLACEMENT_3D('',#15109,#11866,#11867);
#9819=AXIS2_PLACEMENT_3D('',#15110,#11868,#11869);
#9820=AXIS2_PLACEMENT_3D('',#15113,#11872,#11873);
#9821=AXIS2_PLACEMENT_3D('',#15119,#11878,#11879);
#9822=AXIS2_PLACEMENT_3D('',#15122,#11882,#11883);
#9823=AXIS2_PLACEMENT_3D('',#15128,#11888,#11889);
#9824=AXIS2_PLACEMENT_3D('',#15130,#11891,#11892);
#9825=AXIS2_PLACEMENT_3D('',#15131,#11893,#11894);
#9826=AXIS2_PLACEMENT_3D('',#15134,#11896,#11897);
#9827=AXIS2_PLACEMENT_3D('',#15135,#11898,#11899);
#9828=AXIS2_PLACEMENT_3D('',#15136,#11900,#11901);
#9829=AXIS2_PLACEMENT_3D('',#15138,#11902,#11903);
#9830=AXIS2_PLACEMENT_3D('',#15140,#11905,#11906);
#9831=AXIS2_PLACEMENT_3D('',#15142,#11908,#11909);
#9832=AXIS2_PLACEMENT_3D('',#15145,#11912,#11913);
#9833=AXIS2_PLACEMENT_3D('',#15146,#11914,#11915);
#9834=AXIS2_PLACEMENT_3D('',#15148,#11917,#11918);
#9835=AXIS2_PLACEMENT_3D('',#15149,#11919,#11920);
#9836=AXIS2_PLACEMENT_3D('',#15151,#11922,#11923);
#9837=AXIS2_PLACEMENT_3D('',#15152,#11924,#11925);
#9838=AXIS2_PLACEMENT_3D('',#15153,#11926,#11927);
#9839=AXIS2_PLACEMENT_3D('',#15155,#11929,#11930);
#9840=AXIS2_PLACEMENT_3D('',#15156,#11931,#11932);
#9841=AXIS2_PLACEMENT_3D('',#15157,#11933,#11934);
#9842=AXIS2_PLACEMENT_3D('',#15158,#11935,#11936);
#9843=AXIS2_PLACEMENT_3D('',#15161,#11938,#11939);
#9844=AXIS2_PLACEMENT_3D('',#15162,#11940,#11941);
#9845=AXIS2_PLACEMENT_3D('',#15164,#11942,#11943);
#9846=AXIS2_PLACEMENT_3D('',#15165,#11944,#11945);
#11579=DIRECTION('axis',(0.,0.,1.));
#11580=DIRECTION('refdir',(1.,0.,0.));
#11581=DIRECTION('center_axis',(1.,0.,0.));
#11582=DIRECTION('ref_axis',(0.,0.707106781186547,-0.707106781186548));
#11583=DIRECTION('',(0.707106781186548,0.707106781186548,0.));
#11584=DIRECTION('center_axis',(-1.,0.,0.));
#11585=DIRECTION('ref_axis',(0.,0.707106781186547,-0.707106781186548));
#11586=DIRECTION('',(0.707106781186548,0.,-0.707106781186547));
#11587=DIRECTION('center_axis',(1.,0.,0.));
#11588=DIRECTION('ref_axis',(0.,0.707106781186547,-0.707106781186548));
#11589=DIRECTION('center_axis',(-0.707106781186548,0.707106781186548,0.));
#11590=DIRECTION('ref_axis',(0.,0.,1.));
#11591=DIRECTION('',(0.,0.,1.));
#11592=DIRECTION('center_axis',(-0.707106781186548,0.707106781186548,0.));
#11593=DIRECTION('ref_axis',(0.707106781186547,0.707106781186547,0.));
#11594=DIRECTION('',(0.,0.,-1.));
#11595=DIRECTION('center_axis',(1.,0.,0.));
#11596=DIRECTION('ref_axis',(0.,0.,-1.));
#11597=DIRECTION('',(0.,1.,0.));
#11598=DIRECTION('center_axis',(1.,0.,0.));
#11599=DIRECTION('ref_axis',(0.,-0.707106781186547,-0.707106781186548));
#11600=DIRECTION('',(0.,0.,-1.));
#11601=DIRECTION('center_axis',(1.,0.,0.));
#11602=DIRECTION('ref_axis',(0.,0.,-1.));
#11603=DIRECTION('center_axis',(1.,0.,0.));
#11604=DIRECTION('ref_axis',(0.,-0.707106781186547,-0.707106781186548));
#11605=DIRECTION('',(0.707106781186548,0.,-0.707106781186547));
#11606=DIRECTION('center_axis',(-1.,0.,0.));
#11607=DIRECTION('ref_axis',(0.,-0.707106781186547,-0.707106781186548));
#11608=DIRECTION('',(0.707106781186548,-0.707106781186548,0.));
#11609=DIRECTION('center_axis',(-0.707106781186548,0.,-0.707106781186548));
#11610=DIRECTION('ref_axis',(-0.707106781186548,0.,0.707106781186548));
#11611=DIRECTION('',(0.,-1.,0.));
#11612=DIRECTION('center_axis',(1.,0.,0.));
#11613=DIRECTION('ref_axis',(0.,0.707106781186547,0.707106781186548));
#11614=DIRECTION('',(0.707106781186548,0.,0.707106781186547));
#11615=DIRECTION('center_axis',(-1.,0.,0.));
#11616=DIRECTION('ref_axis',(0.,0.707106781186547,0.707106781186548));
#11617=DIRECTION('',(0.707106781186548,0.707106781186548,0.));
#11618=DIRECTION('center_axis',(1.,0.,0.));
#11619=DIRECTION('ref_axis',(0.,0.707106781186547,0.707106781186548));
#11620=DIRECTION('center_axis',(-0.707106781186548,0.,0.707106781186548));
#11621=DIRECTION('ref_axis',(0.707106781186548,0.,0.707106781186548));
#11622=DIRECTION('',(0.,-1.,0.));
#11623=DIRECTION('',(0.707106781186548,0.,0.707106781186547));
#11624=DIRECTION('',(0.,1.,0.));
#11625=DIRECTION('center_axis',(1.,0.,0.));
#11626=DIRECTION('ref_axis',(0.,0.,-1.));
#11627=DIRECTION('',(0.,0.,1.));
#11628=DIRECTION('center_axis',(1.,0.,0.));
#11629=DIRECTION('ref_axis',(0.,0.,-1.));
#11630=DIRECTION('',(0.,0.,-1.));
#11631=DIRECTION('center_axis',(1.,0.,0.));
#11632=DIRECTION('ref_axis',(0.,-0.707106781186547,0.707106781186548));
#11633=DIRECTION('center_axis',(1.,0.,0.));
#11634=DIRECTION('ref_axis',(0.,-0.707106781186547,0.707106781186548));
#11635=DIRECTION('',(0.707106781186548,-0.707106781186548,0.));
#11636=DIRECTION('center_axis',(-1.,0.,0.));
#11637=DIRECTION('ref_axis',(0.,-0.707106781186547,0.707106781186548));
#11638=DIRECTION('center_axis',(-0.707106781186548,-0.707106781186548,0.));
#11639=DIRECTION('ref_axis',(0.,0.,1.));
#11640=DIRECTION('center_axis',(-0.707106781186548,-0.707106781186548,0.));
#11641=DIRECTION('ref_axis',(-0.707106781186547,0.707106781186547,0.));
#11642=DIRECTION('',(0.,0.,1.));
#11643=DIRECTION('',(0.707106781186547,-6.86915450674151E-16,-0.707106781186548));
#11644=DIRECTION('center_axis',(0.,0.,-1.));
#11645=DIRECTION('ref_axis',(1.,0.,0.));
#11646=DIRECTION('',(0.,0.,-1.));
#11647=DIRECTION('center_axis',(1.,0.,0.));
#11648=DIRECTION('ref_axis',(0.,1.,0.));
#11649=DIRECTION('center_axis',(0.707106781186548,0.707106781186548,0.));
#11650=DIRECTION('ref_axis',(-0.707106781186547,0.707106781186547,0.));
#11651=DIRECTION('center_axis',(-0.707106781186548,-0.707106781186548,0.));
#11652=DIRECTION('ref_axis',(-0.707106781186547,0.707106781186547,0.));
#11653=DIRECTION('center_axis',(0.707106781186548,-0.707106781186548,0.));
#11654=DIRECTION('ref_axis',(0.707106781186547,0.707106781186547,0.));
#11655=DIRECTION('center_axis',(1.,0.,0.));
#11656=DIRECTION('ref_axis',(0.,0.,-1.));
#11657=DIRECTION('',(-1.,0.,0.));
#11658=DIRECTION('center_axis',(1.,0.,0.));
#11659=DIRECTION('ref_axis',(0.,0.,-1.));
#11660=DIRECTION('center_axis',(1.,0.,0.));
#11661=DIRECTION('ref_axis',(0.,0.,-1.));
#11662=DIRECTION('center_axis',(0.707106781186548,-0.707106781186548,0.));
#11663=DIRECTION('ref_axis',(0.707106781186547,0.707106781186547,0.));
#11664=DIRECTION('center_axis',(-0.707106781186548,0.707106781186548,0.));
#11665=DIRECTION('ref_axis',(0.707106781186547,0.707106781186547,0.));
#11666=DIRECTION('center_axis',(0.707106781186548,0.707106781186548,0.));
#11667=DIRECTION('ref_axis',(-0.707106781186547,0.707106781186547,0.));
#11668=DIRECTION('center_axis',(1.,0.,0.));
#11669=DIRECTION('ref_axis',(0.,0.,-1.));
#11670=DIRECTION('center_axis',(1.,0.,0.));
#11671=DIRECTION('ref_axis',(0.,0.,-1.));
#11672=DIRECTION('center_axis',(1.,0.,0.));
#11673=DIRECTION('ref_axis',(0.,0.,-1.));
#11674=DIRECTION('center_axis',(-0.707106781186546,0.707106781186549,0.));
#11675=DIRECTION('ref_axis',(-0.707106781186549,-0.707106781186546,0.));
#11676=DIRECTION('',(0.,0.,1.));
#11677=DIRECTION('',(0.,0.,-1.));
#11678=DIRECTION('center_axis',(-0.707106781186545,-0.70710678118655,0.));
#11679=DIRECTION('ref_axis',(0.70710678118655,-0.707106781186545,0.));
#11680=DIRECTION('',(0.,0.,1.));
#11681=DIRECTION('center_axis',(-0.707106781186546,0.707106781186549,0.));
#11682=DIRECTION('ref_axis',(-0.707106781186549,-0.707106781186546,0.));
#11683=DIRECTION('',(0.577350269189626,0.577350269189625,-0.577350269189626));
#11684=DIRECTION('',(0.,0.,1.));
#11685=DIRECTION('',(-0.577350269189626,-0.577350269189625,-0.577350269189626));
#11686=DIRECTION('',(0.,0.,-1.));
#11687=DIRECTION('center_axis',(-0.707106781186546,-0.707106781186549,0.));
#11688=DIRECTION('ref_axis',(0.707106781186549,-0.707106781186546,0.));
#11689=DIRECTION('',(-0.577350269189626,0.577350269189625,0.577350269189626));
#11690=DIRECTION('',(0.,0.,1.));
#11691=DIRECTION('',(0.577350269189626,-0.577350269189625,0.577350269189626));
#11692=DIRECTION('center_axis',(-0.707106781186546,0.707106781186549,0.));
#11693=DIRECTION('ref_axis',(-0.707106781186549,-0.707106781186546,0.));
#11694=DIRECTION('',(0.577350269189627,0.577350269189624,-0.577350269189627));
#11695=DIRECTION('',(0.,0.,1.));
#11696=DIRECTION('',(-0.577350269189627,-0.577350269189624,-0.577350269189627));
#11697=DIRECTION('',(0.,0.,-1.));
#11698=DIRECTION('center_axis',(-0.707106781186546,-0.707106781186549,0.));
#11699=DIRECTION('ref_axis',(0.707106781186549,-0.707106781186546,0.));
#11700=DIRECTION('',(-0.577350269189627,0.577350269189624,0.577350269189627));
#11701=DIRECTION('',(0.,0.,1.));
#11702=DIRECTION('',(0.577350269189626,-0.577350269189624,0.577350269189626));
#11703=DIRECTION('center_axis',(-0.707106781186546,0.707106781186549,0.));
#11704=DIRECTION('ref_axis',(-0.707106781186549,-0.707106781186546,0.));
#11705=DIRECTION('',(0.577350269189627,0.577350269189624,-0.577350269189627));
#11706=DIRECTION('',(0.,0.,1.));
#11707=DIRECTION('',(-0.577350269189627,-0.577350269189624,-0.577350269189627));
#11708=DIRECTION('',(0.,0.,-1.));
#11709=DIRECTION('center_axis',(-0.707106781186546,-0.707106781186549,0.));
#11710=DIRECTION('ref_axis',(0.707106781186549,-0.707106781186546,0.));
#11711=DIRECTION('',(-0.577350269189627,0.577350269189624,0.577350269189627));
#11712=DIRECTION('',(0.,0.,1.));
#11713=DIRECTION('',(0.577350269189627,-0.577350269189624,0.577350269189627));
#11714=DIRECTION('center_axis',(-0.707106781186546,0.707106781186549,0.));
#11715=DIRECTION('ref_axis',(-0.707106781186549,-0.707106781186546,0.));
#11716=DIRECTION('',(0.577350269189626,0.577350269189625,-0.577350269189626));
#11717=DIRECTION('',(0.,0.,1.));
#11718=DIRECTION('',(-0.577350269189626,-0.577350269189625,-0.577350269189626));
#11719=DIRECTION('',(0.,0.,-1.));
#11720=DIRECTION('center_axis',(-0.707106781186546,-0.707106781186549,0.));
#11721=DIRECTION('ref_axis',(0.707106781186549,-0.707106781186546,0.));
#11722=DIRECTION('',(-0.577350269189627,0.577350269189624,0.577350269189627));
#11723=DIRECTION('',(0.,0.,1.));
#11724=DIRECTION('',(0.577350269189627,-0.577350269189624,0.577350269189627));
#11725=DIRECTION('center_axis',(-0.707106781186545,-0.70710678118655,0.));
#11726=DIRECTION('ref_axis',(0.70710678118655,-0.707106781186545,0.));
#11727=DIRECTION('',(0.,0.,1.));
#11728=DIRECTION('',(0.,0.,1.));
#11729=DIRECTION('center_axis',(-0.707106781186546,0.707106781186549,0.));
#11730=DIRECTION('ref_axis',(-0.707106781186549,-0.707106781186546,0.));
#11731=DIRECTION('',(0.,0.,-1.));
#11732=DIRECTION('center_axis',(-0.707106781186546,-0.707106781186549,0.));
#11733=DIRECTION('ref_axis',(0.707106781186549,-0.707106781186546,0.));
#11734=DIRECTION('',(0.,0.,1.));
#11735=DIRECTION('',(0.,0.,1.));
#11736=DIRECTION('center_axis',(-0.707106781186545,0.70710678118655,0.));
#11737=DIRECTION('ref_axis',(-0.70710678118655,-0.707106781186545,0.));
#11738=DIRECTION('',(0.,0.,-1.));
#11739=DIRECTION('center_axis',(-0.707106781186546,0.707106781186549,0.));
#11740=DIRECTION('ref_axis',(-0.707106781186549,-0.707106781186546,0.));
#11741=DIRECTION('',(0.577350269189627,0.577350269189624,-0.577350269189627));
#11742=DIRECTION('',(0.,0.,1.));
#11743=DIRECTION('',(-0.577350269189627,-0.577350269189624,-0.577350269189627));
#11744=DIRECTION('',(0.,0.,-1.));
#11745=DIRECTION('center_axis',(-0.707106781186546,-0.707106781186549,0.));
#11746=DIRECTION('ref_axis',(0.707106781186549,-0.707106781186546,0.));
#11747=DIRECTION('',(-0.577350269189626,0.577350269189625,0.577350269189626));
#11748=DIRECTION('',(0.,0.,1.));
#11749=DIRECTION('',(0.577350269189626,-0.577350269189625,0.577350269189626));
#11750=DIRECTION('center_axis',(-0.707106781186546,0.707106781186549,0.));
#11751=DIRECTION('ref_axis',(-0.707106781186549,-0.707106781186546,0.));
#11752=DIRECTION('',(0.577350269189627,0.577350269189624,-0.577350269189627));
#11753=DIRECTION('',(0.,0.,1.));
#11754=DIRECTION('',(-0.577350269189626,-0.577350269189624,-0.577350269189626));
#11755=DIRECTION('',(0.,0.,-1.));
#11756=DIRECTION('center_axis',(-0.707106781186546,-0.707106781186549,0.));
#11757=DIRECTION('ref_axis',(0.707106781186549,-0.707106781186546,0.));
#11758=DIRECTION('',(-0.577350269189627,0.577350269189624,0.577350269189627));
#11759=DIRECTION('',(0.,0.,1.));
#11760=DIRECTION('',(0.577350269189626,-0.577350269189624,0.577350269189626));
#11761=DIRECTION('center_axis',(-0.707106781186546,-0.707106781186549,0.));
#11762=DIRECTION('ref_axis',(0.707106781186549,-0.707106781186546,0.));
#11763=DIRECTION('',(0.,0.,1.));
#11764=DIRECTION('',(0.,0.,1.));
#11765=DIRECTION('center_axis',(-0.707106781186545,0.70710678118655,0.));
#11766=DIRECTION('ref_axis',(-0.70710678118655,-0.707106781186545,0.));
#11767=DIRECTION('',(0.,0.,-1.));
#11768=DIRECTION('center_axis',(-0.707106781186546,0.707106781186549,0.));
#11769=DIRECTION('ref_axis',(-0.707106781186549,-0.707106781186546,0.));
#11770=DIRECTION('',(0.577350269189626,0.577350269189625,-0.577350269189626));
#11771=DIRECTION('',(0.,0.,1.));
#11772=DIRECTION('',(-0.577350269189626,-0.577350269189625,-0.577350269189626));
#11773=DIRECTION('',(0.,0.,-1.));
#11774=DIRECTION('center_axis',(-0.707106781186546,-0.707106781186549,0.));
#11775=DIRECTION('ref_axis',(0.707106781186549,-0.707106781186546,0.));
#11776=DIRECTION('',(-0.577350269189627,0.577350269189624,0.577350269189627));
#11777=DIRECTION('',(0.,0.,1.));
#11778=DIRECTION('',(0.577350269189627,-0.577350269189624,0.577350269189627));
#11779=DIRECTION('center_axis',(-0.707106781186545,0.70710678118655,0.));
#11780=DIRECTION('ref_axis',(-0.70710678118655,-0.707106781186545,0.));
#11781=DIRECTION('',(0.,0.,1.));
#11782=DIRECTION('',(0.,0.,-1.));
#11783=DIRECTION('center_axis',(-0.707106781186546,-0.707106781186549,0.));
#11784=DIRECTION('ref_axis',(0.707106781186549,-0.707106781186546,0.));
#11785=DIRECTION('',(0.,0.,1.));
#11786=DIRECTION('center_axis',(-0.707106781186546,-0.707106781186549,0.));
#11787=DIRECTION('ref_axis',(0.707106781186549,-0.707106781186546,0.));
#11788=DIRECTION('',(0.,0.,1.));
#11789=DIRECTION('',(0.,0.,1.));
#11790=DIRECTION('center_axis',(-0.707106781186545,0.70710678118655,0.));
#11791=DIRECTION('ref_axis',(-0.70710678118655,-0.707106781186545,0.));
#11792=DIRECTION('',(0.,0.,-1.));
#11793=DIRECTION('center_axis',(-1.,0.,0.));
#11794=DIRECTION('ref_axis',(0.,-0.707106781186547,0.707106781186548));
#11795=DIRECTION('center_axis',(-1.,0.,0.));
#11796=DIRECTION('ref_axis',(0.,-0.707106781186547,0.707106781186548));
#11797=DIRECTION('',(-0.707106781186547,-7.85046229341887E-16,0.707106781186547));
#11798=DIRECTION('center_axis',(1.,0.,0.));
#11799=DIRECTION('ref_axis',(0.,-0.707106781186547,0.707106781186548));
#11800=DIRECTION('',(-0.707106781186547,-0.707106781186547,0.));
#11801=DIRECTION('center_axis',(-1.,0.,0.));
#11802=DIRECTION('ref_axis',(0.,-0.707106781186547,0.707106781186548));
#11803=DIRECTION('center_axis',(-1.,0.,0.));
#11804=DIRECTION('ref_axis',(0.,-0.707106781186547,0.707106781186548));
#11805=DIRECTION('center_axis',(0.707106781186548,0.,0.707106781186548));
#11806=DIRECTION('ref_axis',(0.707106781186548,0.,-0.707106781186548));
#11807=DIRECTION('',(0.,1.,0.));
#11808=DIRECTION('',(-0.707106781186547,0.,0.707106781186547));
#11809=DIRECTION('',(0.,-1.,0.));
#11810=DIRECTION('',(0.,1.,0.));
#11811=DIRECTION('',(0.,1.,0.));
#11812=DIRECTION('',(0.,1.,0.));
#11813=DIRECTION('',(0.,1.,0.));
#11814=DIRECTION('',(0.,1.,0.));
#11815=DIRECTION('',(0.,1.,0.));
#11816=DIRECTION('',(0.,1.,0.));
#11817=DIRECTION('center_axis',(1.,0.,0.));
#11818=DIRECTION('ref_axis',(0.,0.,-1.));
#11819=DIRECTION('center_axis',(-1.,0.,0.));
#11820=DIRECTION('ref_axis',(0.,0.707106781186547,-0.707106781186548));
#11821=DIRECTION('center_axis',(-1.,0.,0.));
#11822=DIRECTION('ref_axis',(0.,0.707106781186547,0.707106781186548));
#11823=DIRECTION('center_axis',(1.,0.,0.));
#11824=DIRECTION('ref_axis',(0.,0.,-1.));
#11825=DIRECTION('',(0.,-1.,0.));
#11826=DIRECTION('center_axis',(-1.,0.,0.));
#11827=DIRECTION('ref_axis',(0.,0.707106781186547,-0.707106781186548));
#11828=DIRECTION('center_axis',(-1.,0.,0.));
#11829=DIRECTION('ref_axis',(0.,0.707106781186547,0.707106781186548));
#11830=DIRECTION('center_axis',(1.,0.,0.));
#11831=DIRECTION('ref_axis',(0.,0.,-1.));
#11832=DIRECTION('',(0.,-1.,0.));
#11833=DIRECTION('center_axis',(1.,0.,0.));
#11834=DIRECTION('ref_axis',(0.,0.,-1.));
#11835=DIRECTION('',(0.,-1.,0.));
#11836=DIRECTION('center_axis',(1.,0.,0.));
#11837=DIRECTION('ref_axis',(0.,0.,-1.));
#11838=DIRECTION('center_axis',(-1.,0.,0.));
#11839=DIRECTION('ref_axis',(0.,-0.707106781186547,-0.707106781186548));
#11840=DIRECTION('center_axis',(1.,0.,0.));
#11841=DIRECTION('ref_axis',(0.,0.,-1.));
#11842=DIRECTION('center_axis',(-1.,0.,0.));
#11843=DIRECTION('ref_axis',(0.,-0.707106781186547,-0.707106781186548));
#11844=DIRECTION('center_axis',(1.,0.,0.));
#11845=DIRECTION('ref_axis',(0.,0.,-1.));
#11846=DIRECTION('center_axis',(-1.,0.,0.));
#11847=DIRECTION('ref_axis',(0.,-0.707106781186547,-0.707106781186548));
#11848=DIRECTION('',(0.,-1.,0.));
#11849=DIRECTION('center_axis',(1.,0.,0.));
#11850=DIRECTION('ref_axis',(0.,0.,-1.));
#11851=DIRECTION('',(0.,-1.,0.));
#11852=DIRECTION('center_axis',(1.,0.,0.));
#11853=DIRECTION('ref_axis',(0.,0.,-1.));
#11854=DIRECTION('',(0.,-1.,0.));
#11855=DIRECTION('center_axis',(1.,0.,0.));
#11856=DIRECTION('ref_axis',(0.,0.,-1.));
#11857=DIRECTION('',(0.,-1.,0.));
#11858=DIRECTION('center_axis',(1.,0.,0.));
#11859=DIRECTION('ref_axis',(0.,0.,-1.));
#11860=DIRECTION('',(0.,-1.,0.));
#11861=DIRECTION('center_axis',(-1.,0.,0.));
#11862=DIRECTION('ref_axis',(0.,0.707106781186547,0.707106781186548));
#11863=DIRECTION('',(-0.707106781186549,0.707106781186546,0.));
#11864=DIRECTION('center_axis',(1.,0.,0.));
#11865=DIRECTION('ref_axis',(0.,0.707106781186547,0.707106781186548));
#11866=DIRECTION('center_axis',(-1.,0.,0.));
#11867=DIRECTION('ref_axis',(0.,0.707106781186547,0.707106781186548));
#11868=DIRECTION('center_axis',(0.707106781186548,-0.707106781186548,0.));
#11869=DIRECTION('ref_axis',(0.,0.,-1.));
#11870=DIRECTION('',(0.,0.,1.));
#11871=DIRECTION('',(0.,0.,-1.));
#11872=DIRECTION('center_axis',(0.,-1.,0.));
#11873=DIRECTION('ref_axis',(0.,0.,-1.));
#11874=DIRECTION('',(0.,0.,1.));
#11875=DIRECTION('',(-1.,0.,0.));
#11876=DIRECTION('',(0.,0.,-1.));
#11877=DIRECTION('',(1.,0.,0.));
#11878=DIRECTION('center_axis',(0.707106781186548,0.707106781186548,0.));
#11879=DIRECTION('ref_axis',(0.,0.,-1.));
#11880=DIRECTION('',(0.,0.,-1.));
#11881=DIRECTION('',(0.,0.,1.));
#11882=DIRECTION('center_axis',(0.,1.,0.));
#11883=DIRECTION('ref_axis',(0.,0.,1.));
#11884=DIRECTION('',(0.,0.,-1.));
#11885=DIRECTION('',(-1.,0.,0.));
#11886=DIRECTION('',(0.,0.,1.));
#11887=DIRECTION('',(1.,0.,0.));
#11888=DIRECTION('center_axis',(1.,0.,0.));
#11889=DIRECTION('ref_axis',(0.,-0.707106781186547,0.707106781186548));
#11890=DIRECTION('',(-1.,0.,0.));
#11891=DIRECTION('center_axis',(-0.707106781186548,-0.707106781186548,0.));
#11892=DIRECTION('ref_axis',(0.,0.,1.));
#11893=DIRECTION('center_axis',(1.,0.,0.));
#11894=DIRECTION('ref_axis',(0.,-0.707106781186547,-0.707106781186548));
#11895=DIRECTION('',(1.,0.,0.));
#11896=DIRECTION('center_axis',(1.,0.,0.));
#11897=DIRECTION('ref_axis',(0.,-0.707106781186547,-0.707106781186548));
#11898=DIRECTION('center_axis',(-0.707106781186548,0.707106781186548,0.));
#11899=DIRECTION('ref_axis',(0.,0.,1.));
#11900=DIRECTION('center_axis',(1.,0.,0.));
#11901=DIRECTION('ref_axis',(0.,0.707106781186547,-0.707106781186548));
#11902=DIRECTION('center_axis',(1.,0.,0.));
#11903=DIRECTION('ref_axis',(0.,0.707106781186547,-0.707106781186548));
#11904=DIRECTION('',(-1.,0.,0.));
#11905=DIRECTION('center_axis',(0.,0.,-1.));
#11906=DIRECTION('ref_axis',(0.,1.,0.));
#11907=DIRECTION('',(0.,1.,0.));
#11908=DIRECTION('center_axis',(-1.,0.,0.));
#11909=DIRECTION('ref_axis',(0.,-0.707106781186547,-0.707106781186548));
#11910=DIRECTION('',(-0.707106781186549,-0.707106781186546,0.));
#11911=DIRECTION('',(0.707106781186547,-7.85046229341887E-16,0.707106781186547));
#11912=DIRECTION('center_axis',(0.707106781186548,-0.707106781186548,0.));
#11913=DIRECTION('ref_axis',(0.,0.,-1.));
#11914=DIRECTION('center_axis',(0.707106781186548,0.707106781186548,0.));
#11915=DIRECTION('ref_axis',(0.,0.,-1.));
#11916=DIRECTION('',(-0.707106781186547,0.707106781186547,0.));
#11917=DIRECTION('center_axis',(-1.,0.,0.));
#11918=DIRECTION('ref_axis',(0.,0.707106781186547,-0.707106781186548));
#11919=DIRECTION('center_axis',(-1.,0.,0.));
#11920=DIRECTION('ref_axis',(0.,0.707106781186547,-0.707106781186548));
#11921=DIRECTION('',(-0.707106781186547,7.85046229341887E-16,-0.707106781186547));
#11922=DIRECTION('center_axis',(0.707106781186548,0.,-0.707106781186548));
#11923=DIRECTION('ref_axis',(-0.707106781186548,0.,-0.707106781186548));
#11924=DIRECTION('center_axis',(1.,0.,0.));
#11925=DIRECTION('ref_axis',(0.,0.,-1.));
#11926=DIRECTION('center_axis',(1.,0.,0.));
#11927=DIRECTION('ref_axis',(0.,0.707106781186547,0.707106781186548));
#11928=DIRECTION('',(1.,0.,0.));
#11929=DIRECTION('center_axis',(0.,0.,1.));
#11930=DIRECTION('ref_axis',(0.,-1.,0.));
#11931=DIRECTION('center_axis',(1.,0.,0.));
#11932=DIRECTION('ref_axis',(0.,0.,-1.));
#11933=DIRECTION('center_axis',(1.,0.,0.));
#11934=DIRECTION('ref_axis',(0.,0.,-1.));
#11935=DIRECTION('center_axis',(1.,0.,0.));
#11936=DIRECTION('ref_axis',(0.,1.,0.));
#11937=DIRECTION('',(-1.,0.,0.));
#11938=DIRECTION('center_axis',(1.,0.,0.));
#11939=DIRECTION('ref_axis',(0.,0.,-1.));
#11940=DIRECTION('center_axis',(-1.,0.,0.));
#11941=DIRECTION('ref_axis',(0.,0.,1.));
#11942=DIRECTION('center_axis',(1.,0.,0.));
#11943=DIRECTION('ref_axis',(0.,0.,-1.));
#11944=DIRECTION('center_axis',(1.,0.,0.));
#11945=DIRECTION('ref_axis',(0.,1.,0.));
#11946=DIRECTION('',(-0.707106781186547,0.707106781186548,8.65956056235494E-17));
#14562=CARTESIAN_POINT('',(0.,0.,0.));
#14563=CARTESIAN_POINT('Origin',(7.25,4.,-14.));
#14564=CARTESIAN_POINT('',(7.,7.5,-14.));
#14565=CARTESIAN_POINT('',(7.5,8.,-14.));
#14566=CARTESIAN_POINT('',(7.25000000000001,7.75000000000001,-14.));
#14567=CARTESIAN_POINT('',(7.5,4.,-18.));
#14568=CARTESIAN_POINT('Origin',(7.5,4.,-14.));
#14569=CARTESIAN_POINT('',(7.,4.,-17.5));
#14570=CARTESIAN_POINT('',(7.25,4.,-17.75));
#14571=CARTESIAN_POINT('Origin',(7.,4.,-14.));
#14572=CARTESIAN_POINT('Origin',(7.25,7.75,-9.));
#14573=CARTESIAN_POINT('',(7.,7.5,-6.61437827766148));
#14574=CARTESIAN_POINT('',(7.,7.5,-9.));
#14575=CARTESIAN_POINT('',(7.5,8.,-6.));
#14576=CARTESIAN_POINT('Origin',(-0.5,0.,0.));
#14577=CARTESIAN_POINT('',(7.5,8.,-9.));
#14578=CARTESIAN_POINT('Origin',(7.,0.,0.));
#14579=CARTESIAN_POINT('',(7.,-4.,-17.5));
#14580=CARTESIAN_POINT('',(7.,-4.,-17.5));
#14581=CARTESIAN_POINT('',(7.,-7.5,-14.));
#14582=CARTESIAN_POINT('Origin',(7.,-4.,-14.));
#14583=CARTESIAN_POINT('',(7.,-7.5,-6.61437827766148));
#14584=CARTESIAN_POINT('',(7.,-7.5,9.));
#14585=CARTESIAN_POINT('Origin',(7.,0.,0.));
#14586=CARTESIAN_POINT('Origin',(7.25,-4.,-14.));
#14587=CARTESIAN_POINT('',(7.5,-4.,-18.));
#14588=CARTESIAN_POINT('',(7.25,-4.,-17.75));
#14589=CARTESIAN_POINT('',(7.5,-8.,-14.));
#14590=CARTESIAN_POINT('Origin',(7.5,-4.,-14.));
#14591=CARTESIAN_POINT('',(7.25000000000001,-7.75000000000001,-14.));
#14592=CARTESIAN_POINT('Origin',(7.25,-4.,-17.75));
#14593=CARTESIAN_POINT('',(7.5,-4.,-18.));
#14594=CARTESIAN_POINT('Origin',(7.25,4.,14.));
#14595=CARTESIAN_POINT('',(7.,4.,17.5));
#14596=CARTESIAN_POINT('',(7.5,4.,18.));
#14597=CARTESIAN_POINT('',(7.25,4.,17.75));
#14598=CARTESIAN_POINT('',(7.5,8.,14.));
#14599=CARTESIAN_POINT('Origin',(7.5,4.,14.));
#14600=CARTESIAN_POINT('',(7.,7.5,14.));
#14601=CARTESIAN_POINT('',(7.25000000000001,7.75000000000001,14.));
#14602=CARTESIAN_POINT('Origin',(7.,4.,14.));
#14603=CARTESIAN_POINT('Origin',(7.25,4.,17.75));
#14604=CARTESIAN_POINT('',(7.,-4.,17.5));
#14605=CARTESIAN_POINT('',(7.,4.,17.5));
#14606=CARTESIAN_POINT('',(7.5,-4.,18.));
#14607=CARTESIAN_POINT('',(7.25,-4.,17.75));
#14608=CARTESIAN_POINT('',(7.5,4.,18.));
#14609=CARTESIAN_POINT('Origin',(7.,0.,0.));
#14610=CARTESIAN_POINT('',(7.,7.5,6.61437827766148));
#14611=CARTESIAN_POINT('',(7.,7.5,-9.));
#14612=CARTESIAN_POINT('',(7.,-7.5,6.61437827766148));
#14613=CARTESIAN_POINT('Origin',(7.,0.,0.));
#14614=CARTESIAN_POINT('',(7.,-7.5,14.));
#14615=CARTESIAN_POINT('',(7.,-7.5,9.));
#14616=CARTESIAN_POINT('Origin',(7.,-4.,14.));
#14617=CARTESIAN_POINT('Origin',(7.25,-4.,14.));
#14618=CARTESIAN_POINT('',(7.5,-8.,14.));
#14619=CARTESIAN_POINT('',(7.25000000000001,-7.75000000000001,14.));
#14620=CARTESIAN_POINT('Origin',(7.5,-4.,14.));
#14621=CARTESIAN_POINT('Origin',(7.25,-7.75,9.));
#14622=CARTESIAN_POINT('',(7.5,-8.,6.));
#14623=CARTESIAN_POINT('Origin',(-0.5,0.,0.));
#14624=CARTESIAN_POINT('',(7.5,-8.,9.));
#14625=CARTESIAN_POINT('Ctrl Pts',(0.95,1.17961196366423E-15,10.));
#14626=CARTESIAN_POINT('Ctrl Pts',(0.95,0.367045949756984,10.));
#14627=CARTESIAN_POINT('Ctrl Pts',(1.07752221450547,0.958324928147939,9.96511377603409));
#14628=CARTESIAN_POINT('Ctrl Pts',(1.50018713245098,1.6077683923816,9.87296307206958));
#14629=CARTESIAN_POINT('Ctrl Pts',(2.00962207364082,2.12638731453228,9.77676926762088));
#14630=CARTESIAN_POINT('Ctrl Pts',(2.93165725867213,2.56177645189286,9.6669255238723));
#14631=CARTESIAN_POINT('Ctrl Pts',(4.07030731706242,2.56318534961883,9.66664213097688));
#14632=CARTESIAN_POINT('Ctrl Pts',(4.98889535650575,2.12294159641258,9.77704450831748));
#14633=CARTESIAN_POINT('Ctrl Pts',(5.50075461569863,1.60769038329482,9.87315468661203));
#14634=CARTESIAN_POINT('Ctrl Pts',(5.92245203441391,0.948791196013554,9.9652950909916));
#14635=CARTESIAN_POINT('Ctrl Pts',(6.13498948573698,0.000273363131113907,
10.0233350886136));
#14636=CARTESIAN_POINT('Ctrl Pts',(5.92374215247507,-0.948040993147089,
9.96567245159996));
#14637=CARTESIAN_POINT('Ctrl Pts',(5.50129034980703,-1.60849172826648,9.87310398731735));
#14638=CARTESIAN_POINT('Ctrl Pts',(4.98823862135932,-2.12213585510122,9.7772258322794));
#14639=CARTESIAN_POINT('Ctrl Pts',(4.07315732767968,-2.56249026452942,9.66671893539352));
#14640=CARTESIAN_POINT('Ctrl Pts',(2.9258047487256,-2.55834406499343,9.66768970154396));
#14641=CARTESIAN_POINT('Ctrl Pts',(1.83672560681065,-2.04463419124632,9.79709054793077));
#14642=CARTESIAN_POINT('Ctrl Pts',(1.13859324782988,-1.16157795697479,9.95148672121565));
#14643=CARTESIAN_POINT('Ctrl Pts',(0.95,-0.367045949756973,10.));
#14644=CARTESIAN_POINT('Ctrl Pts',(0.950000000000001,-1.38777878078145E-16,
10.));
#14645=CARTESIAN_POINT('Ctrl Pts',(1.11666666666667,1.01770443923973E-15,
9.83333333333333));
#14646=CARTESIAN_POINT('Ctrl Pts',(1.11666666666667,0.338138082472203,9.83333333333333));
#14647=CARTESIAN_POINT('Ctrl Pts',(1.23189350754937,0.883178863551863,9.8030072278146));
#14648=CARTESIAN_POINT('Ctrl Pts',(1.62057462760155,1.4901917624257,9.72207568761741));
#14649=CARTESIAN_POINT('Ctrl Pts',(2.09306265257346,1.97974585787698,9.63710887331226));
#14650=CARTESIAN_POINT('Ctrl Pts',(2.96023499641486,2.39843888983004,9.53916716959576));
#14651=CARTESIAN_POINT('Ctrl Pts',(4.04169526814198,2.39979178983521,9.53891552839485));
#14652=CARTESIAN_POINT('Ctrl Pts',(4.90551921769836,1.97654795671124,9.6373419470974));
#14653=CARTESIAN_POINT('Ctrl Pts',(5.38030345361575,1.49011205526117,9.72224154959068));
#14654=CARTESIAN_POINT('Ctrl Pts',(5.76806824424246,0.874302676860821,9.80316241770464));
#14655=CARTESIAN_POINT('Ctrl Pts',(5.96009674079537,0.000236925558889436,
9.85361606443947));
#14656=CARTESIAN_POINT('Ctrl Pts',(5.76921977722431,-0.873560253900129,
9.80348804810433));
#14657=CARTESIAN_POINT('Ctrl Pts',(5.38079732434218,-1.49086268741372,9.72219615790121));
#14658=CARTESIAN_POINT('Ctrl Pts',(4.90485970439378,-1.97578737659674,9.63749666133857));
#14659=CARTESIAN_POINT('Ctrl Pts',(4.04423514273,-2.39913671465528,9.53898427715599));
#14660=CARTESIAN_POINT('Ctrl Pts',(2.95484400730983,-2.39524695639726,9.53982373563105));
#14661=CARTESIAN_POINT('Ctrl Pts',(1.93019347129584,-1.90102207176844,9.65527052164018));
#14662=CARTESIAN_POINT('Ctrl Pts',(1.28758144276905,-1.07065491910773,9.79116853024056));
#14663=CARTESIAN_POINT('Ctrl Pts',(1.11666666666667,-0.338138082472195,
9.83333333333333));
#14664=CARTESIAN_POINT('Ctrl Pts',(1.11666666666667,-1.38777878078145E-16,
9.83333333333333));
#14665=CARTESIAN_POINT('Ctrl Pts',(1.28333333333333,8.55796914815225E-16,
9.66666666666667));
#14666=CARTESIAN_POINT('Ctrl Pts',(1.28333333333333,0.309230215187422,9.66666666666667));
#14667=CARTESIAN_POINT('Ctrl Pts',(1.38626480059327,0.808032798955786,9.64090067959512));
#14668=CARTESIAN_POINT('Ctrl Pts',(1.74096212275212,1.3726151324698,9.57118830316523));
#14669=CARTESIAN_POINT('Ctrl Pts',(2.17650323150611,1.83310440122169,9.49744847900364));
#14670=CARTESIAN_POINT('Ctrl Pts',(2.98881273415759,2.23510132776721,9.41140881531922));
#14671=CARTESIAN_POINT('Ctrl Pts',(4.01308321922153,2.23639823005159,9.41118892581281));
#14672=CARTESIAN_POINT('Ctrl Pts',(4.82214307889098,1.83015431700991,9.49763938587733));
#14673=CARTESIAN_POINT('Ctrl Pts',(5.25985229153288,1.37253372722753,9.57132841256933));
#14674=CARTESIAN_POINT('Ctrl Pts',(5.613684454071,0.799814157708089,9.64102974441768));
#14675=CARTESIAN_POINT('Ctrl Pts',(5.78520399585376,0.000200487986665598,
9.68389704026533));
#14676=CARTESIAN_POINT('Ctrl Pts',(5.61469740197354,-0.799079514653171,
9.6413036446087));
#14677=CARTESIAN_POINT('Ctrl Pts',(5.26030429887732,-1.37323364656096,9.57128832848508));
#14678=CARTESIAN_POINT('Ctrl Pts',(4.82148078742824,-1.82943889809227,9.49776749039775));
#14679=CARTESIAN_POINT('Ctrl Pts',(4.01531295778032,-2.23578316478115,9.41124961891846));
#14680=CARTESIAN_POINT('Ctrl Pts',(2.98388326589406,-2.23214984780108,9.41195776971814));
#14681=CARTESIAN_POINT('Ctrl Pts',(2.02366133578104,-1.75740995229055,9.5134504953496));
#14682=CARTESIAN_POINT('Ctrl Pts',(1.43656963770823,-0.979731881240677,
9.63085033926547));
#14683=CARTESIAN_POINT('Ctrl Pts',(1.28333333333333,-0.309230215187417,
9.66666666666667));
#14684=CARTESIAN_POINT('Ctrl Pts',(1.28333333333333,-1.38777878078145E-16,
9.66666666666667));
#14685=CARTESIAN_POINT('Ctrl Pts',(1.45,6.93889390390723E-16,9.5));
#14686=CARTESIAN_POINT('Ctrl Pts',(1.45,0.280322347902641,9.5));
#14687=CARTESIAN_POINT('Ctrl Pts',(1.54063609363717,0.732886734359709,9.47879413137563));
#14688=CARTESIAN_POINT('Ctrl Pts',(1.86134961790268,1.2550385025139,9.42030091871305));
#14689=CARTESIAN_POINT('Ctrl Pts',(2.25994381043875,1.68646294456639,9.35778808469502));
#14690=CARTESIAN_POINT('Ctrl Pts',(3.01739047190032,2.07176376570438,9.28365046104267));
#14691=CARTESIAN_POINT('Ctrl Pts',(3.98447117030109,2.07300467026798,9.28346232323077));
#14692=CARTESIAN_POINT('Ctrl Pts',(4.73876694008359,1.68376067730857,9.35793682465725));
#14693=CARTESIAN_POINT('Ctrl Pts',(5.13940112945,1.25495539919388,9.42041527554798));
#14694=CARTESIAN_POINT('Ctrl Pts',(5.45930066389954,0.725325638555357,9.47889707113072));
#14695=CARTESIAN_POINT('Ctrl Pts',(5.61031125091214,0.000164050414441131,
9.51417801609118));
#14696=CARTESIAN_POINT('Ctrl Pts',(5.46017502672277,-0.724598775406211,
9.47911924111307));
#14697=CARTESIAN_POINT('Ctrl Pts',(5.13981127341247,-1.2556046057082,9.42038049906894));
#14698=CARTESIAN_POINT('Ctrl Pts',(4.7381018704627,-1.68309041958779,9.35803831945692));
#14699=CARTESIAN_POINT('Ctrl Pts',(3.98639077283064,-2.07242961490702,9.28351496068093));
#14700=CARTESIAN_POINT('Ctrl Pts',(3.01292252447829,-2.06905273920491,9.28409180380522));
#14701=CARTESIAN_POINT('Ctrl Pts',(2.11712920026623,-1.61379783281266,9.37163046905901));
#14702=CARTESIAN_POINT('Ctrl Pts',(1.58555783264741,-0.888808843373621,
9.47053214829039));
#14703=CARTESIAN_POINT('Ctrl Pts',(1.45,-0.280322347902639,9.5));
#14704=CARTESIAN_POINT('Ctrl Pts',(1.45,-1.38777878078145E-16,9.5));
#14705=CARTESIAN_POINT('',(0.950000000000001,-1.38777878078145E-16,10.));
#14706=CARTESIAN_POINT('',(1.45,6.93889390390723E-16,9.5));
#14707=CARTESIAN_POINT('',(0.95,1.17961196366423E-15,10.));
#14708=CARTESIAN_POINT('Ctrl Pts',(1.45,6.93889390390723E-16,9.5));
#14709=CARTESIAN_POINT('Ctrl Pts',(1.45,0.280322347902641,9.5));
#14710=CARTESIAN_POINT('Ctrl Pts',(1.54063609363717,0.732886734359709,9.47879413137563));
#14711=CARTESIAN_POINT('Ctrl Pts',(1.86134961790268,1.2550385025139,9.42030091871305));
#14712=CARTESIAN_POINT('Ctrl Pts',(2.25994381043875,1.68646294456639,9.35778808469502));
#14713=CARTESIAN_POINT('Ctrl Pts',(3.01739047190032,2.07176376570438,9.28365046104267));
#14714=CARTESIAN_POINT('Ctrl Pts',(3.98447117030109,2.07300467026798,9.28346232323077));
#14715=CARTESIAN_POINT('Ctrl Pts',(4.73876694008359,1.68376067730857,9.35793682465725));
#14716=CARTESIAN_POINT('Ctrl Pts',(5.13940112945,1.25495539919388,9.42041527554798));
#14717=CARTESIAN_POINT('Ctrl Pts',(5.45930066389954,0.725325638555357,9.47889707113072));
#14718=CARTESIAN_POINT('Ctrl Pts',(5.61031125091214,0.000164050414441131,
9.51417801609118));
#14719=CARTESIAN_POINT('Ctrl Pts',(5.46017502672277,-0.724598775406211,
9.47911924111307));
#14720=CARTESIAN_POINT('Ctrl Pts',(5.13981127341247,-1.2556046057082,9.42038049906894));
#14721=CARTESIAN_POINT('Ctrl Pts',(4.7381018704627,-1.68309041958779,9.35803831945692));
#14722=CARTESIAN_POINT('Ctrl Pts',(3.98639077283064,-2.07242961490702,9.28351496068093));
#14723=CARTESIAN_POINT('Ctrl Pts',(3.01292252447829,-2.06905273920491,9.28409180380522));
#14724=CARTESIAN_POINT('Ctrl Pts',(2.11712920026623,-1.61379783281266,9.37163046905901));
#14725=CARTESIAN_POINT('Ctrl Pts',(1.58555783264741,-0.888808843373621,
9.47053214829039));
#14726=CARTESIAN_POINT('Ctrl Pts',(1.45,-0.280322347902639,9.5));
#14727=CARTESIAN_POINT('Ctrl Pts',(1.45,-1.38777878078145E-16,9.5));
#14728=CARTESIAN_POINT('Ctrl Pts',(0.950000000000001,-1.38777878078145E-16,
10.));
#14729=CARTESIAN_POINT('Ctrl Pts',(0.95,-0.367045949756973,10.));
#14730=CARTESIAN_POINT('Ctrl Pts',(1.13859324782988,-1.16157795697479,9.95148672121565));
#14731=CARTESIAN_POINT('Ctrl Pts',(1.83672560681065,-2.04463419124632,9.79709054793077));
#14732=CARTESIAN_POINT('Ctrl Pts',(2.9258047487256,-2.55834406499343,9.66768970154396));
#14733=CARTESIAN_POINT('Ctrl Pts',(4.07315732767968,-2.56249026452942,9.66671893539352));
#14734=CARTESIAN_POINT('Ctrl Pts',(4.98823862135932,-2.12213585510122,9.7772258322794));
#14735=CARTESIAN_POINT('Ctrl Pts',(5.50129034980703,-1.60849172826648,9.87310398731735));
#14736=CARTESIAN_POINT('Ctrl Pts',(5.92374215247507,-0.948040993147089,
9.96567245159996));
#14737=CARTESIAN_POINT('Ctrl Pts',(6.13498948573698,0.000273363131113907,
10.0233350886136));
#14738=CARTESIAN_POINT('Ctrl Pts',(5.92245203441391,0.948791196013554,9.9652950909916));
#14739=CARTESIAN_POINT('Ctrl Pts',(5.50075461569863,1.60769038329482,9.87315468661203));
#14740=CARTESIAN_POINT('Ctrl Pts',(4.98889535650575,2.12294159641258,9.77704450831748));
#14741=CARTESIAN_POINT('Ctrl Pts',(4.07030731706242,2.56318534961883,9.66664213097688));
#14742=CARTESIAN_POINT('Ctrl Pts',(2.93165725867213,2.56177645189286,9.6669255238723));
#14743=CARTESIAN_POINT('Ctrl Pts',(2.00962207364082,2.12638731453228,9.77676926762088));
#14744=CARTESIAN_POINT('Ctrl Pts',(1.50018713245098,1.6077683923816,9.87296307206958));
#14745=CARTESIAN_POINT('Ctrl Pts',(1.07752221450547,0.958324928147939,9.96511377603409));
#14746=CARTESIAN_POINT('Ctrl Pts',(0.95,0.367045949756984,10.));
#14747=CARTESIAN_POINT('Ctrl Pts',(0.95,1.17961196366423E-15,10.));
#14748=CARTESIAN_POINT('Origin',(3.5,0.,10.));
#14749=CARTESIAN_POINT('',(1.45,2.64304174990748E-16,5.025));
#14750=CARTESIAN_POINT('',(1.45,2.51052593825207E-16,10.));
#14751=CARTESIAN_POINT('',(3.5,2.05,4.58782355807195));
#14752=CARTESIAN_POINT('Ctrl Pts',(3.5,2.05,4.58782355807195));
#14753=CARTESIAN_POINT('Ctrl Pts',(3.23911658808884,2.05,4.58782355807195));
#14754=CARTESIAN_POINT('Ctrl Pts',(2.96327422636181,1.9972365364845,4.61243172108358));
#14755=CARTESIAN_POINT('Ctrl Pts',(2.4593022166293,1.78717027592319,4.6978188168031));
#14756=CARTESIAN_POINT('Ctrl Pts',(2.23085473008692,1.62999253295176,4.75702184253145));
#14757=CARTESIAN_POINT('Ctrl Pts',(1.87020630601552,1.26934410888037,4.86567773089675));
#14758=CARTESIAN_POINT('Ctrl Pts',(1.71287808635485,1.04082190467728,4.9226508378233));
#14759=CARTESIAN_POINT('Ctrl Pts',(1.50269621880289,0.536556350598789,5.00279010148928));
#14760=CARTESIAN_POINT('Ctrl Pts',(1.45,0.260595900858596,5.025));
#14761=CARTESIAN_POINT('Ctrl Pts',(1.45,4.16333634234434E-16,5.025));
#14762=CARTESIAN_POINT('Ctrl Pts',(1.45,2.77555756156289E-16,5.025));
#14763=CARTESIAN_POINT('Ctrl Pts',(1.45,-0.260595900858595,5.025));
#14764=CARTESIAN_POINT('Ctrl Pts',(1.50269621880289,-0.536556350598789,
5.00279010148928));
#14765=CARTESIAN_POINT('Ctrl Pts',(1.71287808635485,-1.04082190467728,4.9226508378233));
#14766=CARTESIAN_POINT('Ctrl Pts',(1.87020630601552,-1.26934410888037,4.86567773089675));
#14767=CARTESIAN_POINT('Ctrl Pts',(2.23085473008692,-1.62999253295176,4.75702184253145));
#14768=CARTESIAN_POINT('Ctrl Pts',(2.4593022166293,-1.78717027592319,4.6978188168031));
#14769=CARTESIAN_POINT('Ctrl Pts',(2.96327422636181,-1.9972365364845,4.61243172108358));
#14770=CARTESIAN_POINT('Ctrl Pts',(3.23911658808884,-2.05,4.58782355807195));
#14771=CARTESIAN_POINT('Ctrl Pts',(3.76088341191116,-2.05,4.58782355807195));
#14772=CARTESIAN_POINT('Ctrl Pts',(4.03672577363819,-1.9972365364845,4.61243172108358));
#14773=CARTESIAN_POINT('Ctrl Pts',(4.5406977833707,-1.78717027592319,4.6978188168031));
#14774=CARTESIAN_POINT('Ctrl Pts',(4.76914526991308,-1.62999253295176,4.75702184253145));
#14775=CARTESIAN_POINT('Ctrl Pts',(5.12979369398448,-1.26934410888037,4.86567773089675));
#14776=CARTESIAN_POINT('Ctrl Pts',(5.28712191364515,-1.04082190467728,4.9226508378233));
#14777=CARTESIAN_POINT('Ctrl Pts',(5.4973037811971,-0.53655635059879,5.00279010148928));
#14778=CARTESIAN_POINT('Ctrl Pts',(5.55,-0.260595900858596,5.025));
#14779=CARTESIAN_POINT('Ctrl Pts',(5.55,0.260595900858595,5.025));
#14780=CARTESIAN_POINT('Ctrl Pts',(5.4973037811971,0.53655635059879,5.00279010148928));
#14781=CARTESIAN_POINT('Ctrl Pts',(5.28712191364515,1.04082190467728,4.9226508378233));
#14782=CARTESIAN_POINT('Ctrl Pts',(5.12979369398448,1.26934410888037,4.86567773089675));
#14783=CARTESIAN_POINT('Ctrl Pts',(4.76914526991308,1.62999253295176,4.75702184253145));
#14784=CARTESIAN_POINT('Ctrl Pts',(4.5406977833707,1.78717027592319,4.6978188168031));
#14785=CARTESIAN_POINT('Ctrl Pts',(4.03672577363819,1.9972365364845,4.61243172108358));
#14786=CARTESIAN_POINT('Ctrl Pts',(3.76088341191116,2.05,4.58782355807195));
#14787=CARTESIAN_POINT('Ctrl Pts',(3.5,2.05,4.58782355807195));
#14788=CARTESIAN_POINT('Origin',(3.75,0.,0.));
#14789=CARTESIAN_POINT('',(7.,8.5,-5.26782687642637));
#14790=CARTESIAN_POINT('Origin',(15.5,0.,0.));
#14791=CARTESIAN_POINT('',(7.5,-8.,-6.));
#14792=CARTESIAN_POINT('Origin',(-0.5,0.,0.));
#14793=CARTESIAN_POINT('',(7.,-8.5,-5.26782687642637));
#14794=CARTESIAN_POINT('Origin',(15.5,0.,0.));
#14795=CARTESIAN_POINT('',(7.,-10.,-1.22464679914735E-15));
#14796=CARTESIAN_POINT('Origin',(7.,0.,0.));
#14797=CARTESIAN_POINT('',(0.5,-10.,-1.22464679914735E-15));
#14798=CARTESIAN_POINT('',(3.75,-10.,-1.22464679914735E-15));
#14799=CARTESIAN_POINT('Origin',(0.5,0.,0.));
#14800=CARTESIAN_POINT('',(7.,-8.5,5.26782687642637));
#14801=CARTESIAN_POINT('Origin',(7.,0.,0.));
#14802=CARTESIAN_POINT('Origin',(15.5,0.,0.));
#14803=CARTESIAN_POINT('',(7.5,8.,6.));
#14804=CARTESIAN_POINT('Origin',(-0.5,0.,0.));
#14805=CARTESIAN_POINT('',(7.,8.5,5.26782687642637));
#14806=CARTESIAN_POINT('Origin',(15.5,0.,0.));
#14807=CARTESIAN_POINT('Origin',(7.,0.,0.));
#14808=CARTESIAN_POINT('Origin',(12.,0.,0.));
#14809=CARTESIAN_POINT('',(12.,-5.025,-6.15385016571545E-16));
#14810=CARTESIAN_POINT('Origin',(12.,0.,0.));
#14811=CARTESIAN_POINT('Origin',(17.05,6.35,-18.));
#14812=CARTESIAN_POINT('',(16.7,6.,17.2310988842807));
#14813=CARTESIAN_POINT('',(17.,6.3,16.6381811916546));
#14814=CARTESIAN_POINT('Ctrl Pts',(16.7,6.,17.2310988842807));
#14815=CARTESIAN_POINT('Ctrl Pts',(16.865153077165,6.16515307716503,16.9346400379677));
#14816=CARTESIAN_POINT('Ctrl Pts',(17.,6.3,16.6381811916546));
#14817=CARTESIAN_POINT('',(16.7,6.,-17.2310988842807));
#14818=CARTESIAN_POINT('',(16.7,6.,-18.));
#14819=CARTESIAN_POINT('',(17.,6.3,-16.6381811916546));
#14820=CARTESIAN_POINT('Ctrl Pts',(17.,6.3,-16.6381811916546));
#14821=CARTESIAN_POINT('Ctrl Pts',(16.865153077165,6.16515307716504,-16.9346400379676));
#14822=CARTESIAN_POINT('Ctrl Pts',(16.7,6.,-17.2310988842807));
#14823=CARTESIAN_POINT('',(17.,6.3,-9.));
#14824=CARTESIAN_POINT('Origin',(16.7,6.,-18.));
#14825=CARTESIAN_POINT('',(17.,5.7,17.0594117081557));
#14826=CARTESIAN_POINT('Ctrl Pts',(17.,5.7,17.0594117081557));
#14827=CARTESIAN_POINT('Ctrl Pts',(16.8540939564508,5.84590604354921,17.1452552962182));
#14828=CARTESIAN_POINT('Ctrl Pts',(16.7,6.,17.2310988842807));
#14829=CARTESIAN_POINT('',(17.,5.7,-17.0594117081557));
#14830=CARTESIAN_POINT('',(17.,5.7,-9.));
#14831=CARTESIAN_POINT('Ctrl Pts',(16.7,6.,-17.2310988842807));
#14832=CARTESIAN_POINT('Ctrl Pts',(16.8540939564509,5.84590604354905,-17.1452552962181));
#14833=CARTESIAN_POINT('Ctrl Pts',(17.,5.7,-17.0594117081557));
#14834=CARTESIAN_POINT('Origin',(17.05,3.95,-18.));
#14835=CARTESIAN_POINT('',(16.7,3.6,17.8));
#14836=CARTESIAN_POINT('',(17.,3.9,17.5));
#14837=CARTESIAN_POINT('',(22.8666666666667,9.76666666666666,11.6333333333333));
#14838=CARTESIAN_POINT('',(16.7,3.6,-17.8));
#14839=CARTESIAN_POINT('',(16.7,3.6,-18.));
#14840=CARTESIAN_POINT('',(17.,3.9,-17.5));
#14841=CARTESIAN_POINT('',(15.5333333333333,2.43333333333334,-18.9666666666667));
#14842=CARTESIAN_POINT('',(17.,3.9,-9.));
#14843=CARTESIAN_POINT('Origin',(16.7,3.6,-18.));
#14844=CARTESIAN_POINT('',(17.,3.3,17.5));
#14845=CARTESIAN_POINT('',(22.6166666666667,-2.31666666666666,11.8833333333333));
#14846=CARTESIAN_POINT('',(17.,3.3,-17.5));
#14847=CARTESIAN_POINT('',(17.,3.3,-9.));
#14848=CARTESIAN_POINT('',(17.95,2.35000000000001,-16.55));
#14849=CARTESIAN_POINT('Origin',(17.05,1.55,-18.));
#14850=CARTESIAN_POINT('',(16.7,1.2,17.8));
#14851=CARTESIAN_POINT('',(17.,1.5,17.5));
#14852=CARTESIAN_POINT('',(23.2666666666667,7.76666666666666,11.2333333333333));
#14853=CARTESIAN_POINT('',(16.7,1.2,-17.8));
#14854=CARTESIAN_POINT('',(16.7,1.2,-18.));
#14855=CARTESIAN_POINT('',(17.,1.5,-17.5));
#14856=CARTESIAN_POINT('',(15.9333333333333,0.433333333333337,-18.5666666666667));
#14857=CARTESIAN_POINT('',(17.,1.5,-9.));
#14858=CARTESIAN_POINT('Origin',(16.7,1.2,-18.));
#14859=CARTESIAN_POINT('',(17.,0.900000000000001,17.5));
#14860=CARTESIAN_POINT('',(22.2166666666667,-4.31666666666666,12.2833333333333));
#14861=CARTESIAN_POINT('',(17.,0.900000000000001,-17.5));
#14862=CARTESIAN_POINT('',(17.,0.900000000000002,-9.));
#14863=CARTESIAN_POINT('',(17.55,0.350000000000006,-16.95));
#14864=CARTESIAN_POINT('Origin',(17.05,0.349999999999999,-18.));
#14865=CARTESIAN_POINT('',(16.7,-8.88178419700125E-16,17.8));
#14866=CARTESIAN_POINT('',(17.,0.299999999999999,17.5));
#14867=CARTESIAN_POINT('',(23.4666666666667,6.76666666666665,11.0333333333333));
#14868=CARTESIAN_POINT('',(16.7,-8.88178419700125E-16,-17.8));
#14869=CARTESIAN_POINT('',(16.7,-8.88178419700125E-16,-18.));
#14870=CARTESIAN_POINT('',(17.,0.299999999999998,-17.5));
#14871=CARTESIAN_POINT('',(16.1333333333333,-0.566666666666664,-18.3666666666667));
#14872=CARTESIAN_POINT('',(17.,0.299999999999998,-9.));
#14873=CARTESIAN_POINT('Origin',(16.7,-8.88178419700125E-16,-18.));
#14874=CARTESIAN_POINT('',(17.,-0.3,17.5));
#14875=CARTESIAN_POINT('',(22.0166666666667,-5.31666666666666,12.4833333333333));
#14876=CARTESIAN_POINT('',(17.,-0.3,-17.5));
#14877=CARTESIAN_POINT('',(17.,-0.299999999999999,-9.));
#14878=CARTESIAN_POINT('',(17.35,-0.649999999999996,-17.15));
#14879=CARTESIAN_POINT('Origin',(17.05,-2.05,-18.));
#14880=CARTESIAN_POINT('',(16.7,-2.4,17.8));
#14881=CARTESIAN_POINT('',(17.,-2.1,17.5));
#14882=CARTESIAN_POINT('',(23.8666666666667,4.76666666666666,10.6333333333333));
#14883=CARTESIAN_POINT('',(16.7,-2.4,-17.8));
#14884=CARTESIAN_POINT('',(16.7,-2.4,-18.));
#14885=CARTESIAN_POINT('',(17.,-2.1,-17.5));
#14886=CARTESIAN_POINT('',(16.5333333333333,-2.56666666666667,-17.9666666666667));
#14887=CARTESIAN_POINT('',(17.,-2.1,-9.));
#14888=CARTESIAN_POINT('Origin',(16.7,-2.4,-18.));
#14889=CARTESIAN_POINT('',(17.,-2.7,17.5));
#14890=CARTESIAN_POINT('',(21.6166666666667,-7.31666666666666,12.8833333333333));
#14891=CARTESIAN_POINT('',(17.,-2.7,-17.5));
#14892=CARTESIAN_POINT('',(17.,-2.7,-9.));
#14893=CARTESIAN_POINT('',(16.95,-2.65,-17.55));
#14894=CARTESIAN_POINT('Origin',(16.7,-4.8,-18.));
#14895=CARTESIAN_POINT('',(16.7,-4.8,-17.7148351242013));
#14896=CARTESIAN_POINT('',(17.,-5.1,-17.3226495451672));
#14897=CARTESIAN_POINT('Ctrl Pts',(16.7,-4.8,-17.7148351242013));
#14898=CARTESIAN_POINT('Ctrl Pts',(16.8583592135001,-4.95835921350012,-17.5187423346843));
#14899=CARTESIAN_POINT('Ctrl Pts',(17.,-5.1,-17.3226495451672));
#14900=CARTESIAN_POINT('',(16.7,-4.8,17.7148351242013));
#14901=CARTESIAN_POINT('',(16.7,-4.8,-18.));
#14902=CARTESIAN_POINT('',(17.,-5.1,17.3226495451672));
#14903=CARTESIAN_POINT('Ctrl Pts',(17.,-5.1,17.3226495451672));
#14904=CARTESIAN_POINT('Ctrl Pts',(16.8583592135001,-4.95835921350012,17.5187423346843));
#14905=CARTESIAN_POINT('Ctrl Pts',(16.7,-4.8,17.7148351242013));
#14906=CARTESIAN_POINT('',(17.,-5.1,-9.));
#14907=CARTESIAN_POINT('Origin',(17.05,-4.45,-18.));
#14908=CARTESIAN_POINT('',(17.,-4.5,-17.4641016151378));
#14909=CARTESIAN_POINT('Ctrl Pts',(17.,-4.5,-17.4641016151378));
#14910=CARTESIAN_POINT('Ctrl Pts',(16.8552389410473,-4.64476105895267,-17.5894683696695));
#14911=CARTESIAN_POINT('Ctrl Pts',(16.7,-4.8,-17.7148351242013));
#14912=CARTESIAN_POINT('',(17.,-4.5,17.4641016151378));
#14913=CARTESIAN_POINT('',(17.,-4.5,-9.));
#14914=CARTESIAN_POINT('Ctrl Pts',(16.7,-4.8,17.7148351242013));
#14915=CARTESIAN_POINT('Ctrl Pts',(16.8552389410473,-4.64476105895271,17.5894683696695));
#14916=CARTESIAN_POINT('Ctrl Pts',(17.,-4.5,17.4641016151378));
#14917=CARTESIAN_POINT('Origin',(16.7,-6.,-18.));
#14918=CARTESIAN_POINT('',(16.7,-6.,-17.2310988842807));
#14919=CARTESIAN_POINT('',(17.,-6.3,-16.6381811916546));
#14920=CARTESIAN_POINT('Ctrl Pts',(16.7,-6.,-17.2310988842807));
#14921=CARTESIAN_POINT('Ctrl Pts',(16.865153077165,-6.16515307716504,-16.9346400379676));
#14922=CARTESIAN_POINT('Ctrl Pts',(17.,-6.3,-16.6381811916546));
#14923=CARTESIAN_POINT('',(16.7,-6.,17.2310988842807));
#14924=CARTESIAN_POINT('',(16.7,-6.,-18.));
#14925=CARTESIAN_POINT('',(17.,-6.3,16.6381811916546));
#14926=CARTESIAN_POINT('Ctrl Pts',(17.,-6.3,16.6381811916546));
#14927=CARTESIAN_POINT('Ctrl Pts',(16.865153077165,-6.16515307716504,16.9346400379676));
#14928=CARTESIAN_POINT('Ctrl Pts',(16.7,-6.,17.2310988842807));
#14929=CARTESIAN_POINT('',(17.,-6.3,-9.));
#14930=CARTESIAN_POINT('Origin',(17.05,-5.65,-18.));
#14931=CARTESIAN_POINT('',(17.,-5.7,-17.0594117081557));
#14932=CARTESIAN_POINT('Ctrl Pts',(17.,-5.7,-17.0594117081557));
#14933=CARTESIAN_POINT('Ctrl Pts',(16.8540939564507,-5.84590604354931,-17.1452552962182));
#14934=CARTESIAN_POINT('Ctrl Pts',(16.7,-6.,-17.2310988842807));
#14935=CARTESIAN_POINT('',(17.,-5.7,17.0594117081557));
#14936=CARTESIAN_POINT('',(17.,-5.7,-9.));
#14937=CARTESIAN_POINT('Ctrl Pts',(16.7,-6.,17.2310988842807));
#14938=CARTESIAN_POINT('Ctrl Pts',(16.8540939564508,-5.84590604354915,17.1452552962182));
#14939=CARTESIAN_POINT('Ctrl Pts',(17.,-5.7,17.0594117081557));
#14940=CARTESIAN_POINT('Origin',(17.05,-3.25,-18.));
#14941=CARTESIAN_POINT('',(16.7,-3.6,17.8));
#14942=CARTESIAN_POINT('',(17.,-3.3,17.5));
#14943=CARTESIAN_POINT('',(24.0666666666667,3.76666666666665,10.4333333333333));
#14944=CARTESIAN_POINT('',(16.7,-3.6,-17.8));
#14945=CARTESIAN_POINT('',(16.7,-3.6,-18.));
#14946=CARTESIAN_POINT('',(17.,-3.3,-17.5));
#14947=CARTESIAN_POINT('',(16.7333333333333,-3.56666666666667,-17.7666666666667));
#14948=CARTESIAN_POINT('',(17.,-3.3,-9.));
#14949=CARTESIAN_POINT('Origin',(16.7,-3.6,-18.));
#14950=CARTESIAN_POINT('',(17.,-3.9,17.5));
#14951=CARTESIAN_POINT('',(21.4166666666667,-8.31666666666667,13.0833333333333));
#14952=CARTESIAN_POINT('',(17.,-3.9,-17.5));
#14953=CARTESIAN_POINT('',(17.,-3.9,-9.));
#14954=CARTESIAN_POINT('',(16.75,-3.65,-17.75));
#14955=CARTESIAN_POINT('Origin',(17.05,-0.85,-18.));
#14956=CARTESIAN_POINT('',(16.7,-1.2,17.8));
#14957=CARTESIAN_POINT('',(17.,-0.900000000000001,17.5));
#14958=CARTESIAN_POINT('',(23.6666666666667,5.76666666666665,10.8333333333333));
#14959=CARTESIAN_POINT('',(16.7,-1.2,-17.8));
#14960=CARTESIAN_POINT('',(16.7,-1.2,-18.));
#14961=CARTESIAN_POINT('',(17.,-0.900000000000001,-17.5));
#14962=CARTESIAN_POINT('',(16.3333333333333,-1.56666666666667,-18.1666666666667));
#14963=CARTESIAN_POINT('',(17.,-0.900000000000002,-9.));
#14964=CARTESIAN_POINT('Origin',(16.7,-1.2,-18.));
#14965=CARTESIAN_POINT('',(17.,-1.5,17.5));
#14966=CARTESIAN_POINT('',(21.8166666666667,-6.31666666666666,12.6833333333333));
#14967=CARTESIAN_POINT('',(17.,-1.5,-17.5));
#14968=CARTESIAN_POINT('',(17.,-1.5,-9.));
#14969=CARTESIAN_POINT('',(17.15,-1.65,-17.35));
#14970=CARTESIAN_POINT('Origin',(16.7,-7.2,-18.));
#14971=CARTESIAN_POINT('',(16.7,-7.2,-16.0493901531919));
#14972=CARTESIAN_POINT('',(17.,-7.5,-14.));
#14973=CARTESIAN_POINT('Ctrl Pts',(16.7,-7.2,-16.0493901531919));
#14974=CARTESIAN_POINT('Ctrl Pts',(17.,-7.5,-15.024695076596));
#14975=CARTESIAN_POINT('Ctrl Pts',(17.,-7.5,-14.));
#14976=CARTESIAN_POINT('',(16.7,-7.2,16.0493901531919));
#14977=CARTESIAN_POINT('',(16.7,-7.2,-18.));
#14978=CARTESIAN_POINT('',(17.,-7.5,14.));
#14979=CARTESIAN_POINT('Ctrl Pts',(17.,-7.5,14.));
#14980=CARTESIAN_POINT('Ctrl Pts',(17.,-7.5,15.024695076596));
#14981=CARTESIAN_POINT('Ctrl Pts',(16.7,-7.2,16.0493901531919));
#14982=CARTESIAN_POINT('',(17.,-7.5,9.));
#14983=CARTESIAN_POINT('Origin',(17.05,-6.85,-18.));
#14984=CARTESIAN_POINT('',(17.,-6.9,-15.9595917942265));
#14985=CARTESIAN_POINT('Ctrl Pts',(17.,-6.9,-15.9595917942265));
#14986=CARTESIAN_POINT('Ctrl Pts',(16.8533598938642,-7.04664010613577,-16.0044909737091));
#14987=CARTESIAN_POINT('Ctrl Pts',(16.7,-7.2,-16.0493901531919));
#14988=CARTESIAN_POINT('',(17.,-6.9,15.9595917942265));
#14989=CARTESIAN_POINT('',(17.,-6.9,-9.));
#14990=CARTESIAN_POINT('Ctrl Pts',(16.7,-7.2,16.0493901531919));
#14991=CARTESIAN_POINT('Ctrl Pts',(16.8533598938643,-7.04664010613571,16.004490973709));
#14992=CARTESIAN_POINT('Ctrl Pts',(17.,-6.9,15.9595917942265));
#14993=CARTESIAN_POINT('Origin',(17.05,2.75,-18.));
#14994=CARTESIAN_POINT('',(16.7,2.4,17.8));
#14995=CARTESIAN_POINT('',(17.,2.7,17.5));
#14996=CARTESIAN_POINT('',(23.0666666666667,8.76666666666666,11.4333333333333));
#14997=CARTESIAN_POINT('',(16.7,2.4,-17.8));
#14998=CARTESIAN_POINT('',(16.7,2.4,-18.));
#14999=CARTESIAN_POINT('',(17.,2.7,-17.5));
#15000=CARTESIAN_POINT('',(15.7333333333333,1.43333333333334,-18.7666666666667));
#15001=CARTESIAN_POINT('',(17.,2.7,-9.));
#15002=CARTESIAN_POINT('Origin',(16.7,2.4,-18.));
#15003=CARTESIAN_POINT('',(17.,2.1,17.5));
#15004=CARTESIAN_POINT('',(22.4166666666667,-3.31666666666666,12.0833333333333));
#15005=CARTESIAN_POINT('',(17.,2.1,-17.5));
#15006=CARTESIAN_POINT('',(17.,2.1,-9.));
#15007=CARTESIAN_POINT('',(17.75,1.35000000000001,-16.75));
#15008=CARTESIAN_POINT('Origin',(17.05,5.15,-18.));
#15009=CARTESIAN_POINT('',(16.7,4.8,17.7148351242013));
#15010=CARTESIAN_POINT('',(17.,5.1,17.3226495451672));
#15011=CARTESIAN_POINT('Ctrl Pts',(16.7,4.8,17.7148351242013));
#15012=CARTESIAN_POINT('Ctrl Pts',(16.8583592135001,4.95835921350012,17.5187423346843));
#15013=CARTESIAN_POINT('Ctrl Pts',(17.,5.1,17.3226495451672));
#15014=CARTESIAN_POINT('',(16.7,4.8,-17.7148351242013));
#15015=CARTESIAN_POINT('',(16.7,4.8,-18.));
#15016=CARTESIAN_POINT('',(17.,5.1,-17.3226495451672));
#15017=CARTESIAN_POINT('Ctrl Pts',(17.,5.1,-17.3226495451672));
#15018=CARTESIAN_POINT('Ctrl Pts',(16.8583592135001,4.95835921350012,-17.5187423346843));
#15019=CARTESIAN_POINT('Ctrl Pts',(16.7,4.8,-17.7148351242013));
#15020=CARTESIAN_POINT('',(17.,5.1,-9.));
#15021=CARTESIAN_POINT('Origin',(16.7,4.8,-18.));
#15022=CARTESIAN_POINT('',(17.,4.5,17.4641016151378));
#15023=CARTESIAN_POINT('Ctrl Pts',(17.,4.5,17.4641016151378));
#15024=CARTESIAN_POINT('Ctrl Pts',(16.8552389410473,4.64476105895274,17.5894683696696));
#15025=CARTESIAN_POINT('Ctrl Pts',(16.7,4.8,17.7148351242013));
#15026=CARTESIAN_POINT('',(17.,4.5,-17.4641016151378));
#15027=CARTESIAN_POINT('',(17.,4.5,-9.));
#15028=CARTESIAN_POINT('Ctrl Pts',(16.7,4.8,-17.7148351242013));
#15029=CARTESIAN_POINT('Ctrl Pts',(16.8552389410473,4.64476105895272,-17.5894683696695));
#15030=CARTESIAN_POINT('Ctrl Pts',(17.,4.5,-17.4641016151378));
#15031=CARTESIAN_POINT('Origin',(16.7,7.2,-18.));
#15032=CARTESIAN_POINT('',(16.7,7.2,-16.0493901531919));
#15033=CARTESIAN_POINT('',(17.,6.9,-15.9595917942265));
#15034=CARTESIAN_POINT('Ctrl Pts',(16.7,7.2,-16.0493901531919));
#15035=CARTESIAN_POINT('Ctrl Pts',(16.8533598938632,7.04664010613677,-16.0044909737094));
#15036=CARTESIAN_POINT('Ctrl Pts',(17.,6.9,-15.9595917942265));
#15037=CARTESIAN_POINT('',(16.7,7.2,16.0493901531919));
#15038=CARTESIAN_POINT('',(16.7,7.2,-18.));
#15039=CARTESIAN_POINT('',(17.,6.9,15.9595917942265));
#15040=CARTESIAN_POINT('Ctrl Pts',(17.,6.9,15.9595917942265));
#15041=CARTESIAN_POINT('Ctrl Pts',(16.8533598938628,7.04664010613721,16.0044909737095));
#15042=CARTESIAN_POINT('Ctrl Pts',(16.7,7.2,16.0493901531919));
#15043=CARTESIAN_POINT('',(17.,6.9,-9.));
#15044=CARTESIAN_POINT('Origin',(17.05,7.55,-18.));
#15045=CARTESIAN_POINT('',(17.,7.5,-14.));
#15046=CARTESIAN_POINT('Ctrl Pts',(17.,7.5,-14.));
#15047=CARTESIAN_POINT('Ctrl Pts',(17.,7.5,-15.024695076596));
#15048=CARTESIAN_POINT('Ctrl Pts',(16.7,7.2,-16.0493901531919));
#15049=CARTESIAN_POINT('',(17.,7.5,14.));
#15050=CARTESIAN_POINT('',(17.,7.5,-9.));
#15051=CARTESIAN_POINT('Ctrl Pts',(16.7,7.2,16.0493901531919));
#15052=CARTESIAN_POINT('Ctrl Pts',(17.,7.5,15.024695076596));
#15053=CARTESIAN_POINT('Ctrl Pts',(17.,7.5,14.));
#15054=CARTESIAN_POINT('Origin',(16.75,-4.,14.));
#15055=CARTESIAN_POINT('',(17.,-4.,17.5));
#15056=CARTESIAN_POINT('Origin',(17.,-4.,14.));
#15057=CARTESIAN_POINT('',(16.5,-4.,18.));
#15058=CARTESIAN_POINT('',(17.,-4.,17.5));
#15059=CARTESIAN_POINT('',(16.5,-8.,14.));
#15060=CARTESIAN_POINT('Origin',(16.5,-4.,14.));
#15061=CARTESIAN_POINT('',(17.,-7.5,14.));
#15062=CARTESIAN_POINT('Origin',(17.,-4.,14.));
#15063=CARTESIAN_POINT('Origin',(17.,-4.,14.));
#15064=CARTESIAN_POINT('Origin',(16.75,4.,17.75));
#15065=CARTESIAN_POINT('',(17.,4.,17.5));
#15066=CARTESIAN_POINT('',(17.,4.,17.5));
#15067=CARTESIAN_POINT('',(16.5,4.,18.));
#15068=CARTESIAN_POINT('',(17.,4.,17.5));
#15069=CARTESIAN_POINT('',(16.5,4.,18.));
#15070=CARTESIAN_POINT('',(17.,4.,17.5));
#15071=CARTESIAN_POINT('',(17.,4.,17.5));
#15072=CARTESIAN_POINT('',(17.,4.,17.5));
#15073=CARTESIAN_POINT('',(17.,4.,17.5));
#15074=CARTESIAN_POINT('',(17.,4.,17.5));
#15075=CARTESIAN_POINT('',(17.,4.,17.5));
#15076=CARTESIAN_POINT('',(17.,4.,17.5));
#15077=CARTESIAN_POINT('Origin',(17.,0.,0.));
#15078=CARTESIAN_POINT('Origin',(17.,4.,-14.));
#15079=CARTESIAN_POINT('Origin',(17.,4.,14.));
#15080=CARTESIAN_POINT('Origin',(17.,0.,0.));
#15081=CARTESIAN_POINT('',(17.,4.,-17.5));
#15082=CARTESIAN_POINT('',(17.,-4.,-17.5));
#15083=CARTESIAN_POINT('Origin',(17.,4.,-14.));
#15084=CARTESIAN_POINT('Origin',(17.,4.,14.));
#15085=CARTESIAN_POINT('Origin',(17.,0.,0.));
#15086=CARTESIAN_POINT('',(17.,-4.,-17.5));
#15087=CARTESIAN_POINT('Origin',(17.,0.,0.));
#15088=CARTESIAN_POINT('',(17.,-4.,-17.5));
#15089=CARTESIAN_POINT('Origin',(17.,0.,0.));
#15090=CARTESIAN_POINT('Origin',(17.,-4.,-14.));
#15091=CARTESIAN_POINT('Origin',(17.,0.,0.));
#15092=CARTESIAN_POINT('Origin',(17.,-4.,-14.));
#15093=CARTESIAN_POINT('Origin',(17.,0.,0.));
#15094=CARTESIAN_POINT('',(17.,-4.,-17.5));
#15095=CARTESIAN_POINT('Origin',(17.,-4.,-14.));
#15096=CARTESIAN_POINT('',(17.,-4.,-17.5));
#15097=CARTESIAN_POINT('Origin',(17.,0.,0.));
#15098=CARTESIAN_POINT('',(17.,-4.,-17.5));
#15099=CARTESIAN_POINT('Origin',(17.,0.,0.));
#15100=CARTESIAN_POINT('',(17.,-4.,-17.5));
#15101=CARTESIAN_POINT('Origin',(17.,0.,0.));
#15102=CARTESIAN_POINT('',(17.,-4.,-17.5));
#15103=CARTESIAN_POINT('Origin',(17.,0.,0.));
#15104=CARTESIAN_POINT('',(17.,-4.,-17.5));
#15105=CARTESIAN_POINT('Origin',(16.75,4.,14.));
#15106=CARTESIAN_POINT('',(16.5,8.,14.));
#15107=CARTESIAN_POINT('',(17.,7.5,14.));
#15108=CARTESIAN_POINT('Origin',(16.5,4.,14.));
#15109=CARTESIAN_POINT('Origin',(17.,4.,14.));
#15110=CARTESIAN_POINT('Origin',(7.25,-8.25,9.));
#15111=CARTESIAN_POINT('',(7.5,-8.,9.));
#15112=CARTESIAN_POINT('',(7.,-8.5,9.));
#15113=CARTESIAN_POINT('Origin',(7.,-8.,18.));
#15114=CARTESIAN_POINT('',(7.5,-8.,9.));
#15115=CARTESIAN_POINT('',(16.5,-8.,-14.));
#15116=CARTESIAN_POINT('',(7.,-8.,-14.));
#15117=CARTESIAN_POINT('',(16.5,-8.,9.));
#15118=CARTESIAN_POINT('',(7.,-8.,14.));
#15119=CARTESIAN_POINT('Origin',(7.25,8.25,-9.));
#15120=CARTESIAN_POINT('',(7.5,8.,-9.));
#15121=CARTESIAN_POINT('',(7.,8.5,-9.));
#15122=CARTESIAN_POINT('Origin',(7.,8.,-18.));
#15123=CARTESIAN_POINT('',(7.5,8.,-9.));
#15124=CARTESIAN_POINT('',(7.,8.,14.));
#15125=CARTESIAN_POINT('',(16.5,8.,-14.));
#15126=CARTESIAN_POINT('',(16.5,8.,-9.));
#15127=CARTESIAN_POINT('',(7.,8.,-14.));
#15128=CARTESIAN_POINT('Origin',(7.,-4.,14.));
#15129=CARTESIAN_POINT('',(7.,-4.,18.));
#15130=CARTESIAN_POINT('Origin',(7.25,-7.75,9.));
#15131=CARTESIAN_POINT('Origin',(7.,-4.,-14.));
#15132=CARTESIAN_POINT('',(16.5,-4.,-18.));
#15133=CARTESIAN_POINT('',(7.,-4.,-18.));
#15134=CARTESIAN_POINT('Origin',(16.5,-4.,-14.));
#15135=CARTESIAN_POINT('Origin',(7.25,7.75,-9.));
#15136=CARTESIAN_POINT('Origin',(7.,4.,-14.));
#15137=CARTESIAN_POINT('',(16.5,4.,-18.));
#15138=CARTESIAN_POINT('Origin',(16.5,4.,-14.));
#15139=CARTESIAN_POINT('',(7.,4.,-18.));
#15140=CARTESIAN_POINT('Origin',(7.,-8.,-18.));
#15141=CARTESIAN_POINT('',(16.5,-4.,-18.));
#15142=CARTESIAN_POINT('Origin',(16.75,-4.,-14.));
#15143=CARTESIAN_POINT('',(17.,-7.5,-14.));
#15144=CARTESIAN_POINT('',(16.5,-4.,-18.));
#15145=CARTESIAN_POINT('Origin',(16.75,-7.75,9.));
#15146=CARTESIAN_POINT('Origin',(16.75,7.75,-9.));
#15147=CARTESIAN_POINT('',(17.,7.5,-14.));
#15148=CARTESIAN_POINT('Origin',(16.75,4.,-14.));
#15149=CARTESIAN_POINT('Origin',(17.,4.,-14.));
#15150=CARTESIAN_POINT('',(17.,4.,-17.5));
#15151=CARTESIAN_POINT('Origin',(16.75,-4.,-17.75));
#15152=CARTESIAN_POINT('Origin',(17.,0.,0.));
#15153=CARTESIAN_POINT('Origin',(7.,4.,14.));
#15154=CARTESIAN_POINT('',(7.,4.,18.));
#15155=CARTESIAN_POINT('Origin',(7.,8.,18.));
#15156=CARTESIAN_POINT('Origin',(7.,5.025,0.));
#15157=CARTESIAN_POINT('Origin',(7.,5.025,0.));
#15158=CARTESIAN_POINT('Origin',(3.5,0.,0.));
#15159=CARTESIAN_POINT('',(0.,-5.025,-6.15385016571545E-16));
#15160=CARTESIAN_POINT('',(3.5,-5.025,-6.15385016571545E-16));
#15161=CARTESIAN_POINT('Origin',(0.,0.,0.));
#15162=CARTESIAN_POINT('Origin',(0.,9.5,0.));
#15163=CARTESIAN_POINT('',(-2.77555756156289E-16,-9.5,-1.16341445918999E-15));
#15164=CARTESIAN_POINT('Origin',(0.,0.,0.));
#15165=CARTESIAN_POINT('Origin',(0.25,0.,0.));
#15166=CARTESIAN_POINT('',(0.25,-9.75,-1.19403062916867E-15));
#18262=UNCERTAINTY_MEASURE_WITH_UNIT(LENGTH_MEASURE(0.01),#18282,
'DISTANCE_ACCURACY_VALUE',
'Maximum model space distance between geometric entities at asserted c
onnectivities');
#18266=UNCERTAINTY_MEASURE_WITH_UNIT(LENGTH_MEASURE(0.01),#18282,
'DISTANCE_ACCURACY_VALUE',
'Maximum model space distance between geometric entities at asserted c
onnectivities');
#18277=(
GEOMETRIC_REPRESENTATION_CONTEXT(3)
GLOBAL_UNCERTAINTY_ASSIGNED_CONTEXT((#18262))
GLOBAL_UNIT_ASSIGNED_CONTEXT((#18282,#18284,#18285))
REPRESENTATION_CONTEXT('','3D')
);
#18281=(
GEOMETRIC_REPRESENTATION_CONTEXT(3)
GLOBAL_UNCERTAINTY_ASSIGNED_CONTEXT((#18266))
GLOBAL_UNIT_ASSIGNED_CONTEXT((#18282,#18284,#18285))
REPRESENTATION_CONTEXT('','3D')
);
#18282=(
LENGTH_UNIT()
NAMED_UNIT(*)
SI_UNIT(.MILLI.,.METRE.)
);
#18284=(
NAMED_UNIT(*)
PLANE_ANGLE_UNIT()
SI_UNIT($,.RADIAN.)
);
#18285=(
NAMED_UNIT(*)
SI_UNIT($,.STERADIAN.)
SOLID_ANGLE_UNIT()
);
#18296=SHAPE_DEFINITION_REPRESENTATION(#18310,#18348);
#18310=PRODUCT_DEFINITION_SHAPE('',$,#18363);
#18348=SHAPE_REPRESENTATION('',(#9729),#18277);
#18352=PRODUCT_DEFINITION_CONTEXT('part definition',#18396,'design');
#18363=PRODUCT_DEFINITION('2026-10-20-13-03-22-397',
'09_T-Knob_Switch_Handle',#18377,#18352);
#18377=PRODUCT_DEFINITION_FORMATION('',$,#18408);
#18396=APPLICATION_CONTEXT(
'Core Data for Automotive Mechanical Design Process');
#18397=PRODUCT_CONTEXT('part definition',#18396,'mechanical');
#18408=PRODUCT('2026-10-20-13-03-22-397','09_T-Knob_Switch_Handle',$,(#18397));
#18482=COLOUR_RGB('Off White',0.89,0.88,0.83);
#18483=FILL_AREA_STYLE_COLOUR('',#18482);
#18484=FILL_AREA_STYLE('',(#18483));
#18485=SURFACE_STYLE_FILL_AREA(#18484);
#18486=SURFACE_SIDE_STYLE('',(#18485));
#18487=SURFACE_STYLE_USAGE(.BOTH.,#18486);
#18488=PRESENTATION_STYLE_ASSIGNMENT((#18487));
ENDSEC;
END-ISO-10303-21;
